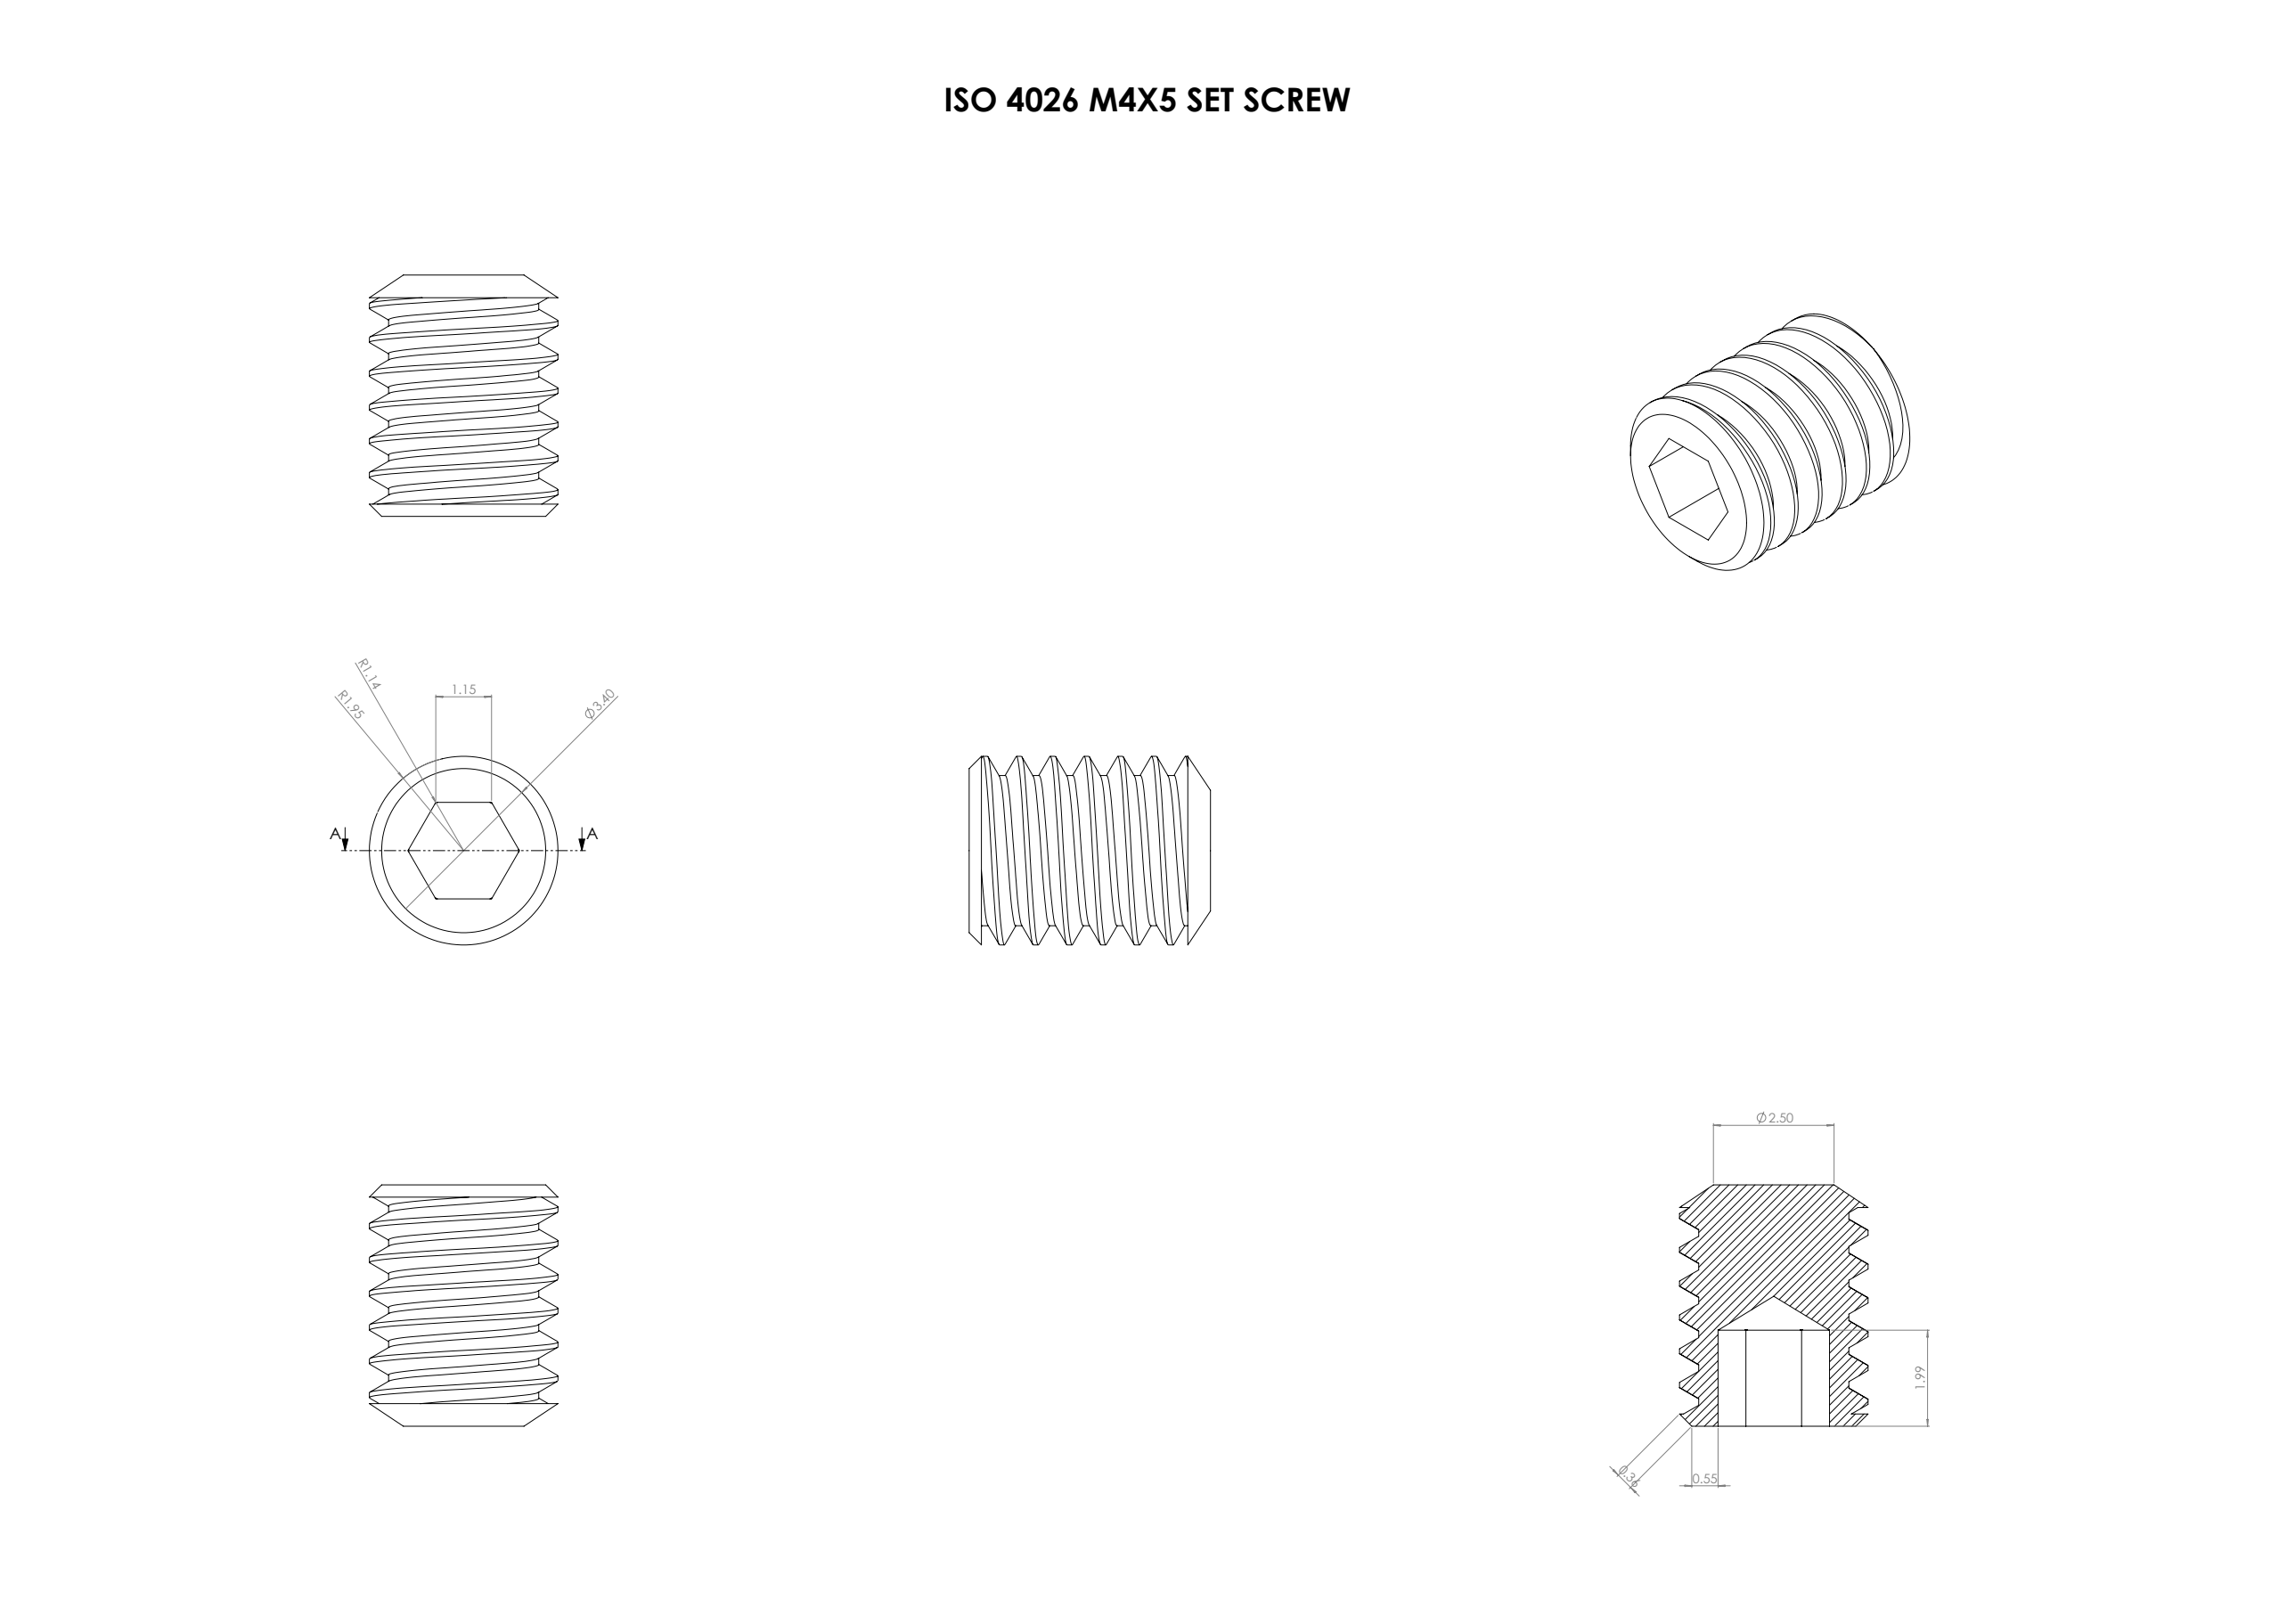
ISO-10303-21;
HEADER;
/* Generated by software containing ST-Developer
 * from STEP Tools, Inc. (www.steptools.com) 
 */

FILE_DESCRIPTION(
/* description */ (''),
/* implementation_level */ '2;1');

FILE_NAME(
/* name */ 
'13_ISO_4026_M4x5_Set_Screw.step',
/* time_stamp */ '2026-10-20T10:06:23-07:00',
/* author */ (''),
/* organization */ (''),
/* preprocessor_version */ 'ST-DEVELOPER v20.2',
/* originating_system */ 'Autodesk Translation Framework v15.15.0.0',
/* authorisation */ '');

FILE_SCHEMA (('AUTOMOTIVE_DESIGN { 1 0 10303 214 3 1 1 }'));
ENDSEC;

DATA;
#10=MECHANICAL_DESIGN_GEOMETRIC_PRESENTATION_REPRESENTATION('',(#466),#38611);
#106=(
BOUNDED_CURVE()
B_SPLINE_CURVE(2,(#25662,#25663,#25664),.UNSPECIFIED.,.F.,.F.)
B_SPLINE_CURVE_WITH_KNOTS((3,3),(0.,0.00350597452849922),.UNSPECIFIED.)
CURVE()
GEOMETRIC_REPRESENTATION_ITEM()
RATIONAL_B_SPLINE_CURVE((1.,1.00010739978215,1.))
REPRESENTATION_ITEM('')
);
#107=(
BOUNDED_CURVE()
B_SPLINE_CURVE(2,(#25666,#25667,#25668),.UNSPECIFIED.,.F.,.F.)
B_SPLINE_CURVE_WITH_KNOTS((3,3),(0.,0.00350597452849927),.UNSPECIFIED.)
CURVE()
GEOMETRIC_REPRESENTATION_ITEM()
RATIONAL_B_SPLINE_CURVE((1.,1.00010739978482,1.))
REPRESENTATION_ITEM('')
);
#108=(
BOUNDED_CURVE()
B_SPLINE_CURVE(2,(#25671,#25672,#25673),.UNSPECIFIED.,.F.,.F.)
B_SPLINE_CURVE_WITH_KNOTS((3,3),(0.,0.0035059745284993),.UNSPECIFIED.)
CURVE()
GEOMETRIC_REPRESENTATION_ITEM()
RATIONAL_B_SPLINE_CURVE((1.,1.00010739978303,1.))
REPRESENTATION_ITEM('')
);
#109=(
BOUNDED_CURVE()
B_SPLINE_CURVE(2,(#25675,#25676,#25677),.UNSPECIFIED.,.F.,.F.)
B_SPLINE_CURVE_WITH_KNOTS((3,3),(0.,0.00350597452849931),.UNSPECIFIED.)
CURVE()
GEOMETRIC_REPRESENTATION_ITEM()
RATIONAL_B_SPLINE_CURVE((1.,1.00010739978394,1.))
REPRESENTATION_ITEM('')
);
#110=(
BOUNDED_CURVE()
B_SPLINE_CURVE(2,(#25680,#25681,#25682),.UNSPECIFIED.,.F.,.F.)
B_SPLINE_CURVE_WITH_KNOTS((3,3),(0.,0.0035059745284993),.UNSPECIFIED.)
CURVE()
GEOMETRIC_REPRESENTATION_ITEM()
RATIONAL_B_SPLINE_CURVE((1.,1.00010739978631,1.))
REPRESENTATION_ITEM('')
);
#111=(
BOUNDED_CURVE()
B_SPLINE_CURVE(2,(#25684,#25685,#25686),.UNSPECIFIED.,.F.,.F.)
B_SPLINE_CURVE_WITH_KNOTS((3,3),(0.,0.00350597452849929),.UNSPECIFIED.)
CURVE()
GEOMETRIC_REPRESENTATION_ITEM()
RATIONAL_B_SPLINE_CURVE((1.,1.00010739978645,1.))
REPRESENTATION_ITEM('')
);
#112=(
BOUNDED_CURVE()
B_SPLINE_CURVE(2,(#25689,#25690,#25691),.UNSPECIFIED.,.F.,.F.)
B_SPLINE_CURVE_WITH_KNOTS((3,3),(0.,0.0035059745284993),.UNSPECIFIED.)
CURVE()
GEOMETRIC_REPRESENTATION_ITEM()
RATIONAL_B_SPLINE_CURVE((1.,1.00010739979569,1.))
REPRESENTATION_ITEM('')
);
#113=(
BOUNDED_CURVE()
B_SPLINE_CURVE(2,(#25693,#25694,#25695),.UNSPECIFIED.,.F.,.F.)
B_SPLINE_CURVE_WITH_KNOTS((3,3),(0.,0.0035059745284993),.UNSPECIFIED.)
CURVE()
GEOMETRIC_REPRESENTATION_ITEM()
RATIONAL_B_SPLINE_CURVE((1.,1.00010739979698,1.))
REPRESENTATION_ITEM('')
);
#114=(
BOUNDED_CURVE()
B_SPLINE_CURVE(2,(#25698,#25699,#25700),.UNSPECIFIED.,.F.,.F.)
B_SPLINE_CURVE_WITH_KNOTS((3,3),(0.,0.00350597452849928),.UNSPECIFIED.)
CURVE()
GEOMETRIC_REPRESENTATION_ITEM()
RATIONAL_B_SPLINE_CURVE((1.,1.00010739978256,1.))
REPRESENTATION_ITEM('')
);
#115=(
BOUNDED_CURVE()
B_SPLINE_CURVE(2,(#25702,#25703,#25704),.UNSPECIFIED.,.F.,.F.)
B_SPLINE_CURVE_WITH_KNOTS((3,3),(0.,0.00350597452849928),.UNSPECIFIED.)
CURVE()
GEOMETRIC_REPRESENTATION_ITEM()
RATIONAL_B_SPLINE_CURVE((1.,1.00010739978752,1.))
REPRESENTATION_ITEM('')
);
#116=(
BOUNDED_CURVE()
B_SPLINE_CURVE(2,(#25707,#25708,#25709),.UNSPECIFIED.,.F.,.F.)
B_SPLINE_CURVE_WITH_KNOTS((3,3),(0.,0.0035059745284993),.UNSPECIFIED.)
CURVE()
GEOMETRIC_REPRESENTATION_ITEM()
RATIONAL_B_SPLINE_CURVE((1.,1.0001073997843,1.))
REPRESENTATION_ITEM('')
);
#117=(
BOUNDED_CURVE()
B_SPLINE_CURVE(2,(#25711,#25712,#25713),.UNSPECIFIED.,.F.,.F.)
B_SPLINE_CURVE_WITH_KNOTS((3,3),(0.,0.00350597452849929),.UNSPECIFIED.)
CURVE()
GEOMETRIC_REPRESENTATION_ITEM()
RATIONAL_B_SPLINE_CURVE((1.,1.00010739978875,1.))
REPRESENTATION_ITEM('')
);
#438=SHAPE_REPRESENTATION_RELATIONSHIP('SRR','None',#38674,#452);
#452=ADVANCED_BREP_SHAPE_REPRESENTATION('',(#480),#38603);
#466=STYLED_ITEM('',(#38885),#480);
#480=MANIFOLD_SOLID_BREP('Set screw',#16240);
#497=B_SPLINE_SURFACE_WITH_KNOTS('',3,3,((#25107,#25108,#25109,#25110,#25111,
#25112,#25113,#25114,#25115,#25116,#25117,#25118,#25119,#25120,#25121,#25122,
#25123,#25124,#25125,#25126,#25127,#25128,#25129,#25130,#25131,#25132,#25133,
#25134,#25135,#25136,#25137,#25138,#25139,#25140,#25141,#25142,#25143,#25144,
#25145,#25146,#25147,#25148,#25149,#25150),(#25151,#25152,#25153,#25154,
#25155,#25156,#25157,#25158,#25159,#25160,#25161,#25162,#25163,#25164,#25165,
#25166,#25167,#25168,#25169,#25170,#25171,#25172,#25173,#25174,#25175,#25176,
#25177,#25178,#25179,#25180,#25181,#25182,#25183,#25184,#25185,#25186,#25187,
#25188,#25189,#25190,#25191,#25192,#25193,#25194),(#25195,#25196,#25197,
#25198,#25199,#25200,#25201,#25202,#25203,#25204,#25205,#25206,#25207,#25208,
#25209,#25210,#25211,#25212,#25213,#25214,#25215,#25216,#25217,#25218,#25219,
#25220,#25221,#25222,#25223,#25224,#25225,#25226,#25227,#25228,#25229,#25230,
#25231,#25232,#25233,#25234,#25235,#25236,#25237,#25238),(#25239,#25240,
#25241,#25242,#25243,#25244,#25245,#25246,#25247,#25248,#25249,#25250,#25251,
#25252,#25253,#25254,#25255,#25256,#25257,#25258,#25259,#25260,#25261,#25262,
#25263,#25264,#25265,#25266,#25267,#25268,#25269,#25270,#25271,#25272,#25273,
#25274,#25275,#25276,#25277,#25278,#25279,#25280,#25281,#25282)),
 .UNSPECIFIED.,.F.,.F.,.F.,(4,4),(4,1,1,1,1,1,1,1,1,1,1,1,1,1,1,1,1,1,1,
1,1,1,1,1,1,1,1,1,1,1,1,1,1,1,1,1,1,1,1,1,1,4),(0.,0.0460148164544132),
(8.31058692273977,9.29723107803592,10.2838752333321,11.2705193886282,12.2571635439244,
13.2438076992205,14.2304518545166,15.2170960098128,16.2037401651089,17.1903843204051,
18.1770284757012,19.1636726309974,20.1503167862935,21.1369609415897,22.1236050968858,
23.110249252182,24.0968934074781,25.0835375627742,26.0701817180704,27.0568258733665,
28.0434700286627,29.0301141839588,30.016758339255,31.0034024945511,31.9900466498473,
32.9766908051434,33.9633349604396,34.9499791157357,35.9366232710318,36.923267426328,
37.9099115816241,38.8965557369203,39.8831998922164,40.8698440475126,41.8564882028087,
42.8431323581049,43.829776513401,44.8164206686971,45.8030648239933,46.7897089792894,
47.7763531345856,48.7629972898817),.UNSPECIFIED.);
#498=B_SPLINE_SURFACE_WITH_KNOTS('',3,3,((#25437,#25438,#25439,#25440,#25441,
#25442,#25443,#25444,#25445,#25446,#25447,#25448,#25449,#25450,#25451,#25452,
#25453,#25454,#25455,#25456,#25457,#25458,#25459,#25460,#25461,#25462,#25463,
#25464,#25465,#25466,#25467,#25468,#25469,#25470,#25471,#25472,#25473,#25474,
#25475,#25476,#25477,#25478,#25479,#25480),(#25481,#25482,#25483,#25484,
#25485,#25486,#25487,#25488,#25489,#25490,#25491,#25492,#25493,#25494,#25495,
#25496,#25497,#25498,#25499,#25500,#25501,#25502,#25503,#25504,#25505,#25506,
#25507,#25508,#25509,#25510,#25511,#25512,#25513,#25514,#25515,#25516,#25517,
#25518,#25519,#25520,#25521,#25522,#25523,#25524),(#25525,#25526,#25527,
#25528,#25529,#25530,#25531,#25532,#25533,#25534,#25535,#25536,#25537,#25538,
#25539,#25540,#25541,#25542,#25543,#25544,#25545,#25546,#25547,#25548,#25549,
#25550,#25551,#25552,#25553,#25554,#25555,#25556,#25557,#25558,#25559,#25560,
#25561,#25562,#25563,#25564,#25565,#25566,#25567,#25568),(#25569,#25570,
#25571,#25572,#25573,#25574,#25575,#25576,#25577,#25578,#25579,#25580,#25581,
#25582,#25583,#25584,#25585,#25586,#25587,#25588,#25589,#25590,#25591,#25592,
#25593,#25594,#25595,#25596,#25597,#25598,#25599,#25600,#25601,#25602,#25603,
#25604,#25605,#25606,#25607,#25608,#25609,#25610,#25611,#25612)),
 .UNSPECIFIED.,.F.,.F.,.F.,(4,4),(4,1,1,1,1,1,1,1,1,1,1,1,1,1,1,1,1,1,1,
1,1,1,1,1,1,1,1,1,1,1,1,1,1,1,1,1,1,1,1,1,1,4),(0.,0.0460148164544132),
(11.6154215191106,12.6020656744068,13.5887098297029,14.5753539849991,15.5619981402952,
16.5486422955914,17.5352864508875,18.5219306061837,19.5085747614798,20.4952189167759,
21.4818630720721,22.4685072273682,23.4551513826644,24.4417955379605,25.4284396932567,
26.4150838485528,27.401728003849,28.3883721591451,29.3750163144413,30.3616604697374,
31.3483046250335,32.3349487803297,33.3215929356258,34.308237090922,35.2948812462181,
36.2815254015143,37.2681695568104,38.2548137121066,39.2414578674027,40.2281020226988,
41.214746177995,42.2013903332911,43.1880344885873,44.1746786438834,45.1613227991796,
46.1479669544757,47.1346111097719,48.121255265068,49.1078994203642,50.0945435756603,
51.0811877309565,52.0678318862526),.UNSPECIFIED.);
#560=B_SPLINE_CURVE_WITH_KNOTS('',3,(#24587,#24588,#24589,#24590,#24591,
#24592,#24593,#24594,#24595,#24596),.UNSPECIFIED.,.F.,.F.,(4,3,3,4),(-4.09254174883832,
-3.94657662118458,-2.95993246588844,-2.06514013327811),.UNSPECIFIED.);
#561=B_SPLINE_CURVE_WITH_KNOTS('',3,(#24599,#24600,#24601,#24602,#24603,
#24604,#24605),.UNSPECIFIED.,.F.,.F.,(4,3,4),(0.,0.986644155296146,1.11419103802958),
 .UNSPECIFIED.);
#562=B_SPLINE_CURVE_WITH_KNOTS('',3,(#24610,#24611,#24612,#24613,#24614,
#24615,#24616,#24617,#24618,#24619,#24620,#24621,#24622,#24623,#24624,#24625,
#24626,#24627,#24628,#24629,#24630,#24631),.UNSPECIFIED.,.F.,.F.,(4,3,3,
3,3,3,3,4),(-10.3757270560179,-9.86644155296145,-8.87979739766531,-7.89315324236916,
-6.90650908707302,-5.91986493177687,-4.93322077648073,-4.09254174883832),
 .UNSPECIFIED.);
#563=B_SPLINE_CURVE_WITH_KNOTS('',3,(#24632,#24633,#24634,#24635,#24636,
#24637,#24638,#24639,#24640,#24641,#24642,#24643,#24644,#24645,#24646,#24647,
#24648,#24649,#24650,#24651,#24652,#24653),.UNSPECIFIED.,.F.,.F.,(4,3,3,
3,3,3,3,4),(1.11419103802958,1.97328831059229,2.95993246588844,3.94657662118458,
4.93322077648073,5.91986493177687,6.90650908707302,7.39737634520917),
 .UNSPECIFIED.);
#564=B_SPLINE_CURVE_WITH_KNOTS('',3,(#24658,#24659,#24660,#24661,#24662,
#24663,#24664,#24665,#24666,#24667,#24668,#24669,#24670,#24671,#24672,#24673,
#24674,#24675,#24676,#24677,#24678,#24679),.UNSPECIFIED.,.F.,.F.,(4,3,3,
3,3,3,3,4),(-16.6589123631975,-15.7863064847383,-14.7996623294422,-13.813018174146,
-12.8263740188499,-11.8397298635537,-10.8530857082576,-10.3757270560179),
 .UNSPECIFIED.);
#565=B_SPLINE_CURVE_WITH_KNOTS('',3,(#24680,#24681,#24682,#24683,#24684,
#24685,#24686,#24687,#24688,#24689,#24690,#24691,#24692,#24693,#24694,#24695,
#24696,#24697,#24698,#24699,#24700,#24701),.UNSPECIFIED.,.F.,.F.,(4,3,3,
3,3,3,3,4),(7.39737634520917,7.89315324236916,8.87979739766531,9.86644155296146,
10.8530857082576,11.8397298635537,12.8263740188499,13.6805616523888),
 .UNSPECIFIED.);
#566=B_SPLINE_CURVE_WITH_KNOTS('',3,(#24706,#24707,#24708,#24709,#24710,
#24711,#24712,#24713,#24714,#24715,#24716,#24717,#24718,#24719,#24720,#24721,
#24722,#24723,#24724,#24725,#24726,#24727,#24728,#24729,#24730),
 .UNSPECIFIED.,.F.,.F.,(4,3,3,3,3,3,3,3,4),(-22.9420976703771,-22.6928155718113,
-21.7061714165152,-20.719527261219,-19.7328831059229,-18.7462389506268,
-17.7595947953306,-16.7729506400345,-16.6589123631975),.UNSPECIFIED.);
#567=B_SPLINE_CURVE_WITH_KNOTS('',3,(#24731,#24732,#24733,#24734,#24735,
#24736,#24737,#24738,#24739,#24740,#24741,#24742,#24743,#24744,#24745,#24746,
#24747,#24748,#24749,#24750,#24751,#24752,#24753,#24754,#24755),
 .UNSPECIFIED.,.F.,.F.,(4,3,3,3,3,3,3,3,4),(13.6805616523888,13.813018174146,
14.7996623294422,15.7863064847383,16.7729506400345,17.7595947953306,18.7462389506268,
19.7328831059229,19.9637469595683),.UNSPECIFIED.);
#568=B_SPLINE_CURVE_WITH_KNOTS('',3,(#24760,#24761,#24762,#24763,#24764,
#24765,#24766,#24767,#24768,#24769,#24770,#24771,#24772,#24773,#24774,#24775,
#24776,#24777,#24778,#24779,#24780,#24781),.UNSPECIFIED.,.F.,.F.,(4,3,3,
3,3,3,3,4),(-29.2252829775567,-28.6126805035882,-27.6260363482921,-26.6393921929959,
-25.6527480376998,-24.6661038824036,-23.6794597271075,-22.9420976703771),
 .UNSPECIFIED.);
#569=B_SPLINE_CURVE_WITH_KNOTS('',3,(#24782,#24783,#24784,#24785,#24786,
#24787,#24788,#24789,#24790,#24791,#24792,#24793,#24794,#24795,#24796,#24797,
#24798,#24799,#24800,#24801,#24802,#24803),.UNSPECIFIED.,.F.,.F.,(4,3,3,
3,3,3,3,4),(19.9637469595683,20.719527261219,21.7061714165152,22.6928155718113,
23.6794597271075,24.6661038824036,25.6527480376998,26.2469322667479),
 .UNSPECIFIED.);
#570=B_SPLINE_CURVE_WITH_KNOTS('',3,(#24808,#24809,#24810,#24811,#24812,
#24813,#24814,#24815,#24816,#24817,#24818,#24819,#24820,#24821,#24822,#24823,
#24824,#24825,#24826,#24827,#24828,#24829),.UNSPECIFIED.,.F.,.F.,(4,3,3,
3,3,3,3,4),(-35.5084682847363,-34.5325454353651,-33.5459012800689,-32.5592571247728,
-31.5726129694767,-30.5859688141805,-29.5993246588844,-29.2252829775567),
 .UNSPECIFIED.);
#571=B_SPLINE_CURVE_WITH_KNOTS('',3,(#24830,#24831,#24832,#24833,#24834,
#24835,#24836,#24837,#24838,#24839,#24840,#24841,#24842,#24843,#24844,#24845,
#24846,#24847,#24848,#24849,#24850,#24851),.UNSPECIFIED.,.F.,.F.,(4,3,3,
3,3,3,3,4),(26.2469322667479,26.6393921929959,27.6260363482921,28.6126805035882,
29.5993246588844,30.5859688141805,31.5726129694767,32.5301175739275),
 .UNSPECIFIED.);
#572=B_SPLINE_CURVE_WITH_KNOTS('',3,(#24857,#24858,#24859,#24860,#24861,
#24862,#24863),.UNSPECIFIED.,.F.,.F.,(4,1,1,1,4),(47.1238898038469,47.1346111097719,
48.121255265068,49.1078994203642,50.0026917529745),.UNSPECIFIED.);
#573=B_SPLINE_CURVE_WITH_KNOTS('',3,(#24866,#24867,#24868,#24869,#24870),
 .UNSPECIFIED.,.F.,.F.,(4,1,4),(47.1238898038469,47.7763531345856,48.7629972898817),
 .UNSPECIFIED.);
#574=B_SPLINE_CURVE_WITH_KNOTS('',3,(#24875,#24876,#24877,#24878,#24879,
#24880,#24881,#24882,#24883,#24884),.UNSPECIFIED.,.F.,.F.,(4,1,1,1,1,1,
1,4),(40.8407044966673,41.214746177995,42.2013903332911,43.1880344885873,
44.1746786438834,45.1613227991796,46.1479669544757,47.1238898038469),
 .UNSPECIFIED.);
#575=B_SPLINE_CURVE_WITH_KNOTS('',3,(#24885,#24886,#24887,#24888,#24889,
#24890,#24891,#24892,#24893,#24894,#24895),.UNSPECIFIED.,.F.,.F.,(4,1,1,
1,1,1,1,1,4),(40.8407044966673,40.8698440475126,41.8564882028087,42.8431323581049,
43.829776513401,44.8164206686971,45.8030648239933,46.7897089792894,47.1238898038469),
 .UNSPECIFIED.);
#576=B_SPLINE_CURVE_WITH_KNOTS('',3,(#24900,#24901,#24902,#24903,#24904,
#24905,#24906,#24907,#24908,#24909),.UNSPECIFIED.,.F.,.F.,(4,1,1,1,1,1,
1,4),(34.5575191894877,35.2948812462181,36.2815254015143,37.2681695568104,
38.2548137121066,39.2414578674027,40.2281020226988,40.8407044966673),
 .UNSPECIFIED.);
#577=B_SPLINE_CURVE_WITH_KNOTS('',3,(#24910,#24911,#24912,#24913,#24914,
#24915,#24916,#24917,#24918,#24919),.UNSPECIFIED.,.F.,.F.,(4,1,1,1,1,1,
1,4),(34.5575191894877,34.9499791157357,35.9366232710318,36.923267426328,
37.9099115816241,38.8965557369203,39.8831998922164,40.8407044966673),
 .UNSPECIFIED.);
#578=B_SPLINE_CURVE_WITH_KNOTS('',3,(#24924,#24925,#24926,#24927,#24928,
#24929,#24930,#24931,#24932,#24933,#24934),.UNSPECIFIED.,.F.,.F.,(4,1,1,
1,1,1,1,1,4),(28.2743338823081,28.3883721591451,29.3750163144413,30.3616604697374,
31.3483046250335,32.3349487803297,33.3215929356258,34.308237090922,34.5575191894877),
 .UNSPECIFIED.);
#579=B_SPLINE_CURVE_WITH_KNOTS('',3,(#24935,#24936,#24937,#24938,#24939,
#24940,#24941,#24942,#24943,#24944),.UNSPECIFIED.,.F.,.F.,(4,1,1,1,1,1,
1,4),(28.2743338823081,29.0301141839588,30.016758339255,31.0034024945511,
31.9900466498473,32.9766908051434,33.9633349604396,34.5575191894877),
 .UNSPECIFIED.);
#580=B_SPLINE_CURVE_WITH_KNOTS('',3,(#24949,#24950,#24951,#24952,#24953,
#24954,#24955,#24956,#24957,#24958),.UNSPECIFIED.,.F.,.F.,(4,1,1,1,1,1,
1,4),(21.9911485751285,22.4685072273682,23.4551513826644,24.4417955379605,
25.4284396932567,26.4150838485528,27.401728003849,28.2743338823081),
 .UNSPECIFIED.);
#581=B_SPLINE_CURVE_WITH_KNOTS('',3,(#24959,#24960,#24961,#24962,#24963,
#24964,#24965,#24966,#24967,#24968,#24969),.UNSPECIFIED.,.F.,.F.,(4,1,1,
1,1,1,1,1,4),(21.9911485751285,22.1236050968858,23.110249252182,24.0968934074781,
25.0835375627742,26.0701817180704,27.0568258733665,28.0434700286627,28.2743338823081),
 .UNSPECIFIED.);
#582=B_SPLINE_CURVE_WITH_KNOTS('',3,(#24974,#24975,#24976,#24977,#24978,
#24979,#24980,#24981,#24982,#24983),.UNSPECIFIED.,.F.,.F.,(4,1,1,1,1,1,
1,4),(15.707963267949,16.5486422955914,17.5352864508875,18.5219306061837,
19.5085747614798,20.4952189167759,21.4818630720721,21.9911485751285),
 .UNSPECIFIED.);
#583=B_SPLINE_CURVE_WITH_KNOTS('',3,(#24984,#24985,#24986,#24987,#24988,
#24989,#24990,#24991,#24992,#24993),.UNSPECIFIED.,.F.,.F.,(4,1,1,1,1,1,
1,4),(15.7079632679489,16.2037401651089,17.1903843204051,18.1770284757012,
19.1636726309974,20.1503167862935,21.1369609415897,21.9911485751285),
 .UNSPECIFIED.);
#584=B_SPLINE_CURVE_WITH_KNOTS('',3,(#24996,#24997,#24998,#24999,#25000,
#25001,#25002,#25003,#25004,#25005,#25006,#25007,#25008,#25009,#25010,#25011,
#25012,#25013,#25014,#25015,#25016,#25017,#25018,#25019,#25020,#25021,#25022,
#25023,#25024,#25025,#25026,#25027,#25028,#25029,#25030,#25031,#25032,#25033,
#25034,#25035,#25036,#25037,#25038,#25039,#25040,#25041,#25042,#25043,#25044,
#25045,#25046,#25047),.UNSPECIFIED.,.F.,.F.,(4,3,3,3,3,3,3,3,3,3,3,3,3,
3,3,3,3,4),(-0.366397579005847,-0.351842688178875,-0.332838158855069,-0.315678481693382,
-0.289420321645097,-0.273011785342624,-0.237897749313856,-0.221715923866805,
-0.207723971026893,-0.185180840167277,-0.161636550067305,-0.147128811889025,
-0.135731814711402,-0.101798861033552,-0.076880688176872,-0.0670092782892109,
-0.0285139790106868,0.),.UNSPECIFIED.);
#585=B_SPLINE_CURVE_WITH_KNOTS('',3,(#25052,#25053,#25054,#25055,#25056,
#25057,#25058,#25059,#25060,#25061,#25062,#25063,#25064,#25065,#25066,#25067,
#25068,#25069,#25070,#25071,#25072,#25073,#25074,#25075,#25076,#25077,#25078,
#25079,#25080,#25081,#25082,#25083,#25084,#25085,#25086,#25087,#25088,#25089,
#25090,#25091,#25092,#25093,#25094,#25095,#25096,#25097,#25098,#25099,#25100,
#25101,#25102,#25103,#25104,#25105,#25106),.UNSPECIFIED.,.F.,.F.,(4,3,3,
3,3,3,3,3,3,3,3,3,3,3,3,3,3,3,4),(-0.364629307890685,-0.346730130939237,
-0.318258076668756,-0.304671300367645,-0.283283926727407,-0.268750032662776,
-0.256211185988777,-0.219678588916904,-0.20148985221534,-0.1862389075973,
-0.164290383513372,-0.139072476943319,-0.127435374126706,-0.116240718055298,
-0.0871805385414733,-0.0683502117761216,-0.0546744719449251,-0.022336513706662,
0.),.UNSPECIFIED.);
#586=B_SPLINE_CURVE_WITH_KNOTS('',3,(#25283,#25284,#25285,#25286,#25287,
#25288,#25289,#25290,#25291,#25292,#25293,#25294,#25295,#25296,#25297,#25298,
#25299,#25300,#25301,#25302,#25303,#25304),.UNSPECIFIED.,.F.,.F.,(4,3,3,
3,3,3,3,4),(32.5301175739275,32.5592571247728,33.5459012800689,34.5325454353651,
35.5191895906612,36.5058337459574,37.4924779012535,38.3872702338639),
 .UNSPECIFIED.);
#587=B_SPLINE_CURVE_WITH_KNOTS('',3,(#25306,#25307,#25308,#25309,#25310,
#25311,#25312,#25313,#25314,#25315,#25316,#25317,#25318,#25319,#25320,#25321,
#25322,#25323,#25324,#25325,#25326,#25327,#25328,#25329,#25330,#25331,#25332,
#25333,#25334,#25335,#25336,#25337,#25338,#25339,#25340,#25341,#25342,#25343,
#25344,#25345,#25346,#25347,#25348,#25349,#25350,#25351,#25352,#25353,#25354,
#25355,#25356,#25357),.UNSPECIFIED.,.F.,.F.,(4,3,3,3,3,3,3,3,3,3,3,3,3,
3,3,3,3,4),(-0.36639757900584,-0.351842688178868,-0.332838163030847,-0.315678486081905,
-0.289414746484995,-0.273012692426124,-0.237898677161377,-0.221717024761523,
-0.207724021339265,-0.18518084016727,-0.161636547239729,-0.147128781690345,
-0.135731805846515,-0.101798854384886,-0.0768806612204703,-0.0670092358876265,
-0.0285139219945927,0.),.UNSPECIFIED.);
#588=B_SPLINE_CURVE_WITH_KNOTS('',3,(#25358,#25359,#25360,#25361,#25362,
#25363,#25364,#25365,#25366),.UNSPECIFIED.,.F.,.F.,(4,1,1,1,1,1,4),(10.3757270560179,
11.2705193886282,12.2571635439244,13.2438076992205,14.2304518545166,15.2170960098128,
15.7079632679489),.UNSPECIFIED.);
#589=B_SPLINE_CURVE_WITH_KNOTS('',3,(#25372,#25373,#25374,#25375,#25376,
#25377,#25378,#25379,#25380,#25381,#25382,#25383,#25384,#25385,#25386,#25387,
#25388,#25389,#25390,#25391,#25392,#25393,#25394,#25395,#25396,#25397,#25398,
#25399,#25400,#25401,#25402,#25403,#25404,#25405,#25406,#25407,#25408,#25409,
#25410,#25411,#25412,#25413,#25414,#25415,#25416,#25417,#25418,#25419,#25420,
#25421,#25422,#25423,#25424,#25425,#25426),.UNSPECIFIED.,.F.,.F.,(4,3,3,
3,3,3,3,3,3,3,3,3,3,3,3,3,3,3,4),(-0.36462930789067,-0.346730130939223,
-0.318258061840929,-0.304671288555113,-0.283283871503023,-0.268749409502959,
-0.256211230718671,-0.219678613621225,-0.201489854814136,-0.186238903270344,
-0.164290383513369,-0.139072549937506,-0.127435742460392,-0.116240765389693,
-0.0871805740422699,-0.0683502946375612,-0.0546744738896406,-0.0223365680991636,
0.),.UNSPECIFIED.);
#590=B_SPLINE_CURVE_WITH_KNOTS('',3,(#25429,#25430,#25431,#25432,#25433,
#25434,#25435,#25436),.UNSPECIFIED.,.F.,.F.,(4,1,1,1,1,4),(11.6154215191106,
12.6020656744068,13.5887098297029,14.5753539849991,15.5619981402952,15.707963267949),
 .UNSPECIFIED.);
#591=B_SPLINE_CURVE_WITH_KNOTS('',3,(#25613,#25614,#25615,#25616,#25617,
#25618,#25619,#25620,#25621,#25622,#25623,#25624,#25625,#25626,#25627,#25628,
#25629,#25630,#25631),.UNSPECIFIED.,.F.,.F.,(4,3,3,3,3,3,4),(-40.452410367142,
-39.4657662118458,-38.4791220565497,-37.4924779012535,-36.5058337459574,
-35.5191895906612,-35.5084682847363),.UNSPECIFIED.);
#916=CYLINDRICAL_SURFACE('',#16835,0.1954);
#917=CYLINDRICAL_SURFACE('',#16837,0.1954);
#918=CYLINDRICAL_SURFACE('',#16838,0.1954);
#919=CYLINDRICAL_SURFACE('',#16839,0.1954);
#920=CYLINDRICAL_SURFACE('',#16840,0.1954);
#921=CYLINDRICAL_SURFACE('',#16841,0.1954);
#922=CYLINDRICAL_SURFACE('',#16842,0.15555);
#923=CYLINDRICAL_SURFACE('',#16844,0.15555);
#924=CYLINDRICAL_SURFACE('',#16845,0.15555);
#925=CYLINDRICAL_SURFACE('',#16846,0.15555);
#926=CYLINDRICAL_SURFACE('',#16847,0.15555);
#927=CYLINDRICAL_SURFACE('',#16848,0.15555);
#928=CYLINDRICAL_SURFACE('',#16856,0.15555);
#929=CYLINDRICAL_SURFACE('',#16904,0.1954);
#1186=FACE_BOUND('',#3044,.T.);
#1363=CIRCLE('',#16836,0.1954);
#1364=CIRCLE('',#16843,0.15555);
#1365=CIRCLE('',#16850,0.1954);
#1366=CIRCLE('',#16851,0.1954);
#1367=CIRCLE('',#16853,0.1954);
#1368=CIRCLE('',#16854,0.1954);
#1369=CIRCLE('',#16855,0.15555);
#1370=CIRCLE('',#16858,0.115470053837925);
#1371=CIRCLE('',#16860,0.115470053837925);
#1372=CIRCLE('',#16862,0.115470053837925);
#1373=CIRCLE('',#16864,0.115470053837925);
#1374=CIRCLE('',#16866,0.115470053837925);
#1375=CIRCLE('',#16868,0.115470053837925);
#1376=CIRCLE('',#16870,0.113827101150665);
#1377=CIRCLE('',#16871,0.113827101150665);
#1378=CIRCLE('',#16872,0.113827101150665);
#1379=CIRCLE('',#16873,0.113827101150665);
#1380=CIRCLE('',#16874,0.113827101150665);
#1381=CIRCLE('',#16875,0.113827101150665);
#1382=CIRCLE('',#16876,0.113827101150665);
#1383=CIRCLE('',#16902,0.125);
#1384=CIRCLE('',#16905,0.1954);
#1385=CIRCLE('',#16907,0.17);
#1740=CONICAL_SURFACE('',#16869,0.0577350269189626,1.02403331474479);
#1741=CONICAL_SURFACE('',#16903,0.1625,0.982793723247329);
#1742=CONICAL_SURFACE('',#16906,0.185,0.785398163397449);
#2047=FACE_OUTER_BOUND('',#2991,.T.);
#2048=FACE_OUTER_BOUND('',#2992,.T.);
#2049=FACE_OUTER_BOUND('',#2993,.T.);
#2050=FACE_OUTER_BOUND('',#2994,.T.);
#2051=FACE_OUTER_BOUND('',#2995,.T.);
#2052=FACE_OUTER_BOUND('',#2996,.T.);
#2053=FACE_OUTER_BOUND('',#2997,.T.);
#2054=FACE_OUTER_BOUND('',#2998,.T.);
#2055=FACE_OUTER_BOUND('',#2999,.T.);
#2056=FACE_OUTER_BOUND('',#3000,.T.);
#2057=FACE_OUTER_BOUND('',#3001,.T.);
#2058=FACE_OUTER_BOUND('',#3002,.T.);
#2059=FACE_OUTER_BOUND('',#3003,.T.);
#2060=FACE_OUTER_BOUND('',#3004,.T.);
#2061=FACE_OUTER_BOUND('',#3005,.T.);
#2062=FACE_OUTER_BOUND('',#3006,.T.);
#2063=FACE_OUTER_BOUND('',#3007,.T.);
#2064=FACE_OUTER_BOUND('',#3008,.T.);
#2065=FACE_OUTER_BOUND('',#3009,.T.);
#2066=FACE_OUTER_BOUND('',#3010,.T.);
#2067=FACE_OUTER_BOUND('',#3011,.T.);
#2068=FACE_OUTER_BOUND('',#3012,.T.);
#2069=FACE_OUTER_BOUND('',#3013,.T.);
#2070=FACE_OUTER_BOUND('',#3014,.T.);
#2071=FACE_OUTER_BOUND('',#3015,.T.);
#2072=FACE_OUTER_BOUND('',#3016,.T.);
#2073=FACE_OUTER_BOUND('',#3017,.T.);
#2074=FACE_OUTER_BOUND('',#3018,.T.);
#2075=FACE_OUTER_BOUND('',#3019,.T.);
#2076=FACE_OUTER_BOUND('',#3020,.T.);
#2077=FACE_OUTER_BOUND('',#3021,.T.);
#2078=FACE_OUTER_BOUND('',#3022,.T.);
#2079=FACE_OUTER_BOUND('',#3023,.T.);
#2080=FACE_OUTER_BOUND('',#3024,.T.);
#2081=FACE_OUTER_BOUND('',#3025,.T.);
#2082=FACE_OUTER_BOUND('',#3026,.T.);
#2083=FACE_OUTER_BOUND('',#3027,.T.);
#2084=FACE_OUTER_BOUND('',#3028,.T.);
#2085=FACE_OUTER_BOUND('',#3029,.T.);
#2086=FACE_OUTER_BOUND('',#3030,.T.);
#2087=FACE_OUTER_BOUND('',#3031,.T.);
#2088=FACE_OUTER_BOUND('',#3032,.T.);
#2089=FACE_OUTER_BOUND('',#3033,.T.);
#2090=FACE_OUTER_BOUND('',#3034,.T.);
#2091=FACE_OUTER_BOUND('',#3035,.T.);
#2092=FACE_OUTER_BOUND('',#3036,.T.);
#2093=FACE_OUTER_BOUND('',#3037,.T.);
#2094=FACE_OUTER_BOUND('',#3038,.T.);
#2095=FACE_OUTER_BOUND('',#3039,.T.);
#2096=FACE_OUTER_BOUND('',#3040,.T.);
#2097=FACE_OUTER_BOUND('',#3041,.T.);
#2098=FACE_OUTER_BOUND('',#3042,.T.);
#2099=FACE_OUTER_BOUND('',#3043,.T.);
#2991=EDGE_LOOP('',(#11365,#11366,#11367,#11368));
#2992=EDGE_LOOP('',(#11369,#11370,#11371,#11372));
#2993=EDGE_LOOP('',(#11373,#11374,#11375,#11376));
#2994=EDGE_LOOP('',(#11377,#11378,#11379,#11380));
#2995=EDGE_LOOP('',(#11381,#11382,#11383,#11384));
#2996=EDGE_LOOP('',(#11385,#11386,#11387,#11388));
#2997=EDGE_LOOP('',(#11389,#11390,#11391,#11392));
#2998=EDGE_LOOP('',(#11393,#11394,#11395,#11396));
#2999=EDGE_LOOP('',(#11397,#11398,#11399,#11400));
#3000=EDGE_LOOP('',(#11401,#11402,#11403,#11404));
#3001=EDGE_LOOP('',(#11405,#11406,#11407,#11408));
#3002=EDGE_LOOP('',(#11409,#11410,#11411,#11412));
#3003=EDGE_LOOP('',(#11413,#11414,#11415,#11416,#11417));
#3004=EDGE_LOOP('',(#11418,#11419,#11420,#11421,#11422,#11423,#11424,#11425,
#11426,#11427,#11428,#11429,#11430,#11431,#11432,#11433));
#3005=EDGE_LOOP('',(#11434,#11435,#11436,#11437,#11438));
#3006=EDGE_LOOP('',(#11439,#11440,#11441,#11442));
#3007=EDGE_LOOP('',(#11443,#11444,#11445,#11446,#11447,#11448,#11449,#11450,
#11451,#11452,#11453,#11454,#11455,#11456,#11457,#11458));
#3008=EDGE_LOOP('',(#11459,#11460));
#3009=EDGE_LOOP('',(#11461,#11462));
#3010=EDGE_LOOP('',(#11463,#11464));
#3011=EDGE_LOOP('',(#11465,#11466));
#3012=EDGE_LOOP('',(#11467,#11468));
#3013=EDGE_LOOP('',(#11469,#11470));
#3014=EDGE_LOOP('',(#11471,#11472,#11473,#11474,#11475,#11476,#11477,#11478,
#11479,#11480,#11481,#11482,#11483,#11484,#11485,#11486,#11487,#11488,#11489,
#11490,#11491,#11492,#11493,#11494,#11495,#11496,#11497));
#3015=EDGE_LOOP('',(#11498,#11499,#11500,#11501));
#3016=EDGE_LOOP('',(#11502,#11503,#11504));
#3017=EDGE_LOOP('',(#11505,#11506,#11507,#11508));
#3018=EDGE_LOOP('',(#11509,#11510,#11511));
#3019=EDGE_LOOP('',(#11512,#11513,#11514));
#3020=EDGE_LOOP('',(#11515,#11516,#11517,#11518));
#3021=EDGE_LOOP('',(#11519,#11520,#11521));
#3022=EDGE_LOOP('',(#11522,#11523,#11524,#11525));
#3023=EDGE_LOOP('',(#11526,#11527,#11528));
#3024=EDGE_LOOP('',(#11529,#11530,#11531));
#3025=EDGE_LOOP('',(#11532,#11533,#11534));
#3026=EDGE_LOOP('',(#11535,#11536,#11537));
#3027=EDGE_LOOP('',(#11538,#11539,#11540));
#3028=EDGE_LOOP('',(#11541,#11542,#11543));
#3029=EDGE_LOOP('',(#11544,#11545,#11546));
#3030=EDGE_LOOP('',(#11547,#11548,#11549,#11550));
#3031=EDGE_LOOP('',(#11551,#11552,#11553,#11554));
#3032=EDGE_LOOP('',(#11555,#11556,#11557));
#3033=EDGE_LOOP('',(#11558,#11559,#11560));
#3034=EDGE_LOOP('',(#11561,#11562,#11563));
#3035=EDGE_LOOP('',(#11564,#11565,#11566,#11567));
#3036=EDGE_LOOP('',(#11568,#11569,#11570));
#3037=EDGE_LOOP('',(#11571,#11572,#11573));
#3038=EDGE_LOOP('',(#11574,#11575,#11576));
#3039=EDGE_LOOP('',(#11577));
#3040=EDGE_LOOP('',(#11578,#11579,#11580,#11581,#11582,#11583));
#3041=EDGE_LOOP('',(#11584,#11585,#11586,#11587));
#3042=EDGE_LOOP('',(#11588,#11589,#11590,#11591,#11592,#11593));
#3043=EDGE_LOOP('',(#11594));
#3044=EDGE_LOOP('',(#11595,#11596,#11597,#11598,#11599,#11600));
#4111=LINE('',#24585,#5335);
#4112=LINE('',#24609,#5336);
#4113=LINE('',#24657,#5337);
#4114=LINE('',#24705,#5338);
#4115=LINE('',#24759,#5339);
#4116=LINE('',#24807,#5340);
#4117=LINE('',#24855,#5341);
#4118=LINE('',#24874,#5342);
#4119=LINE('',#24899,#5343);
#4120=LINE('',#24923,#5344);
#4121=LINE('',#24948,#5345);
#4122=LINE('',#24973,#5346);
#4123=LINE('',#25635,#5347);
#4124=LINE('',#25639,#5348);
#4125=LINE('',#25643,#5349);
#4126=LINE('',#25647,#5350);
#4127=LINE('',#25651,#5351);
#4128=LINE('',#25654,#5352);
#4129=LINE('',#25659,#5353);
#4130=LINE('',#25717,#5354);
#4131=LINE('',#25719,#5355);
#4132=LINE('',#25720,#5356);
#4133=LINE('',#25723,#5357);
#4134=LINE('',#25724,#5358);
#4135=LINE('',#25727,#5359);
#4136=LINE('',#25728,#5360);
#4137=LINE('',#25731,#5361);
#4138=LINE('',#25732,#5362);
#4139=LINE('',#25735,#5363);
#4140=LINE('',#25736,#5364);
#4141=LINE('',#25739,#5365);
#4142=LINE('',#25740,#5366);
#4143=LINE('',#25743,#5367);
#4144=LINE('',#25744,#5368);
#4145=LINE('',#25747,#5369);
#4146=LINE('',#25748,#5370);
#4147=LINE('',#25751,#5371);
#4148=LINE('',#25752,#5372);
#4149=LINE('',#25754,#5373);
#4150=LINE('',#25756,#5374);
#4151=LINE('',#25759,#5375);
#4152=LINE('',#25762,#5376);
#4153=LINE('',#25763,#5377);
#4154=LINE('',#25765,#5378);
#4155=LINE('',#25767,#5379);
#4156=LINE('',#25770,#5380);
#4157=LINE('',#25771,#5381);
#4158=LINE('',#25773,#5382);
#4159=LINE('',#25777,#5383);
#4160=LINE('',#25785,#5384);
#4161=LINE('',#25791,#5385);
#5335=VECTOR('',#19128,0.2);
#5336=VECTOR('',#19133,0.2);
#5337=VECTOR('',#19136,0.2);
#5338=VECTOR('',#19139,0.2);
#5339=VECTOR('',#19142,0.2);
#5340=VECTOR('',#19145,0.2);
#5341=VECTOR('',#19148,0.15555);
#5342=VECTOR('',#19153,0.15555);
#5343=VECTOR('',#19156,0.15555);
#5344=VECTOR('',#19159,0.15555);
#5345=VECTOR('',#19162,0.15555);
#5346=VECTOR('',#19165,0.15555);
#5347=VECTOR('',#19184,1.);
#5348=VECTOR('',#19189,1.);
#5349=VECTOR('',#19194,1.);
#5350=VECTOR('',#19199,1.);
#5351=VECTOR('',#19204,1.);
#5352=VECTOR('',#19209,1.);
#5353=VECTOR('',#19214,0.0577350269189626);
#5354=VECTOR('',#19231,1.);
#5355=VECTOR('',#19232,1.);
#5356=VECTOR('',#19233,1.);
#5357=VECTOR('',#19236,1.);
#5358=VECTOR('',#19237,1.);
#5359=VECTOR('',#19240,1.);
#5360=VECTOR('',#19241,1.);
#5361=VECTOR('',#19244,1.);
#5362=VECTOR('',#19245,1.);
#5363=VECTOR('',#19248,1.);
#5364=VECTOR('',#19249,1.);
#5365=VECTOR('',#19252,1.);
#5366=VECTOR('',#19253,1.);
#5367=VECTOR('',#19256,1.);
#5368=VECTOR('',#19257,1.);
#5369=VECTOR('',#19260,1.);
#5370=VECTOR('',#19261,1.);
#5371=VECTOR('',#19264,1.);
#5372=VECTOR('',#19265,1.);
#5373=VECTOR('',#19268,1.);
#5374=VECTOR('',#19271,1.);
#5375=VECTOR('',#19276,1.);
#5376=VECTOR('',#19279,1.);
#5377=VECTOR('',#19280,1.);
#5378=VECTOR('',#19283,1.);
#5379=VECTOR('',#19286,1.);
#5380=VECTOR('',#19289,1.);
#5381=VECTOR('',#19290,1.);
#5382=VECTOR('',#19293,1.);
#5383=VECTOR('',#19300,1.);
#5384=VECTOR('',#19313,0.1625);
#5385=VECTOR('',#19322,0.185);
#6521=VERTEX_POINT('',#24583);
#6522=VERTEX_POINT('',#24584);
#6523=VERTEX_POINT('',#24586);
#6524=VERTEX_POINT('',#24597);
#6525=VERTEX_POINT('',#24607);
#6526=VERTEX_POINT('',#24608);
#6527=VERTEX_POINT('',#24655);
#6528=VERTEX_POINT('',#24656);
#6529=VERTEX_POINT('',#24703);
#6530=VERTEX_POINT('',#24704);
#6531=VERTEX_POINT('',#24757);
#6532=VERTEX_POINT('',#24758);
#6533=VERTEX_POINT('',#24805);
#6534=VERTEX_POINT('',#24806);
#6535=VERTEX_POINT('',#24853);
#6536=VERTEX_POINT('',#24854);
#6537=VERTEX_POINT('',#24856);
#6538=VERTEX_POINT('',#24864);
#6539=VERTEX_POINT('',#24872);
#6540=VERTEX_POINT('',#24873);
#6541=VERTEX_POINT('',#24897);
#6542=VERTEX_POINT('',#24898);
#6543=VERTEX_POINT('',#24921);
#6544=VERTEX_POINT('',#24922);
#6545=VERTEX_POINT('',#24946);
#6546=VERTEX_POINT('',#24947);
#6547=VERTEX_POINT('',#24971);
#6548=VERTEX_POINT('',#24972);
#6549=VERTEX_POINT('',#24995);
#6550=VERTEX_POINT('',#25048);
#6551=VERTEX_POINT('',#25050);
#6552=VERTEX_POINT('',#25305);
#6553=VERTEX_POINT('',#25368);
#6554=VERTEX_POINT('',#25371);
#6555=VERTEX_POINT('',#25633);
#6556=VERTEX_POINT('',#25634);
#6557=VERTEX_POINT('',#25638);
#6558=VERTEX_POINT('',#25642);
#6559=VERTEX_POINT('',#25646);
#6560=VERTEX_POINT('',#25650);
#6561=VERTEX_POINT('',#25657);
#6562=VERTEX_POINT('',#25658);
#6563=VERTEX_POINT('',#25660);
#6564=VERTEX_POINT('',#25665);
#6565=VERTEX_POINT('',#25669);
#6566=VERTEX_POINT('',#25674);
#6567=VERTEX_POINT('',#25678);
#6568=VERTEX_POINT('',#25683);
#6569=VERTEX_POINT('',#25687);
#6570=VERTEX_POINT('',#25692);
#6571=VERTEX_POINT('',#25696);
#6572=VERTEX_POINT('',#25701);
#6573=VERTEX_POINT('',#25705);
#6574=VERTEX_POINT('',#25710);
#6575=VERTEX_POINT('',#25716);
#6576=VERTEX_POINT('',#25718);
#6577=VERTEX_POINT('',#25722);
#6578=VERTEX_POINT('',#25726);
#6579=VERTEX_POINT('',#25730);
#6580=VERTEX_POINT('',#25734);
#6581=VERTEX_POINT('',#25738);
#6582=VERTEX_POINT('',#25742);
#6583=VERTEX_POINT('',#25746);
#6584=VERTEX_POINT('',#25750);
#6585=VERTEX_POINT('',#25761);
#6586=VERTEX_POINT('',#25769);
#6587=VERTEX_POINT('',#25782);
#6588=VERTEX_POINT('',#25789);
#8298=EDGE_CURVE('',#6521,#6522,#4111,.T.);
#8299=EDGE_CURVE('',#6521,#6523,#560,.T.);
#8300=EDGE_CURVE('',#6523,#6524,#1363,.T.);
#8301=EDGE_CURVE('',#6524,#6522,#561,.T.);
#8302=EDGE_CURVE('',#6525,#6526,#4112,.T.);
#8303=EDGE_CURVE('',#6525,#6521,#562,.T.);
#8304=EDGE_CURVE('',#6522,#6526,#563,.T.);
#8305=EDGE_CURVE('',#6527,#6528,#4113,.T.);
#8306=EDGE_CURVE('',#6527,#6525,#564,.T.);
#8307=EDGE_CURVE('',#6526,#6528,#565,.T.);
#8308=EDGE_CURVE('',#6529,#6530,#4114,.T.);
#8309=EDGE_CURVE('',#6529,#6527,#566,.T.);
#8310=EDGE_CURVE('',#6528,#6530,#567,.T.);
#8311=EDGE_CURVE('',#6531,#6532,#4115,.T.);
#8312=EDGE_CURVE('',#6531,#6529,#568,.T.);
#8313=EDGE_CURVE('',#6530,#6532,#569,.T.);
#8314=EDGE_CURVE('',#6533,#6534,#4116,.T.);
#8315=EDGE_CURVE('',#6533,#6531,#570,.T.);
#8316=EDGE_CURVE('',#6532,#6534,#571,.T.);
#8317=EDGE_CURVE('',#6535,#6536,#4117,.T.);
#8318=EDGE_CURVE('',#6535,#6537,#572,.T.);
#8319=EDGE_CURVE('',#6538,#6537,#1364,.T.);
#8320=EDGE_CURVE('',#6536,#6538,#573,.T.);
#8321=EDGE_CURVE('',#6539,#6540,#4118,.T.);
#8322=EDGE_CURVE('',#6539,#6535,#574,.T.);
#8323=EDGE_CURVE('',#6540,#6536,#575,.T.);
#8324=EDGE_CURVE('',#6541,#6542,#4119,.T.);
#8325=EDGE_CURVE('',#6541,#6539,#576,.T.);
#8326=EDGE_CURVE('',#6542,#6540,#577,.T.);
#8327=EDGE_CURVE('',#6543,#6544,#4120,.T.);
#8328=EDGE_CURVE('',#6543,#6541,#578,.T.);
#8329=EDGE_CURVE('',#6544,#6542,#579,.T.);
#8330=EDGE_CURVE('',#6545,#6546,#4121,.T.);
#8331=EDGE_CURVE('',#6545,#6543,#580,.T.);
#8332=EDGE_CURVE('',#6546,#6544,#581,.T.);
#8333=EDGE_CURVE('',#6547,#6548,#4122,.T.);
#8334=EDGE_CURVE('',#6547,#6545,#582,.T.);
#8335=EDGE_CURVE('',#6548,#6546,#583,.T.);
#8336=EDGE_CURVE('',#6537,#6549,#584,.T.);
#8337=EDGE_CURVE('',#6550,#6549,#1365,.F.);
#8338=EDGE_CURVE('',#6551,#6550,#1366,.F.);
#8339=EDGE_CURVE('',#6551,#6538,#585,.T.);
#8340=EDGE_CURVE('',#6534,#6551,#586,.T.);
#8341=EDGE_CURVE('',#6552,#6524,#587,.T.);
#8342=EDGE_CURVE('',#6552,#6548,#588,.T.);
#8343=EDGE_CURVE('',#6524,#6553,#1367,.T.);
#8344=EDGE_CURVE('',#6553,#6523,#1368,.T.);
#8345=EDGE_CURVE('',#6523,#6554,#589,.T.);
#8346=EDGE_CURVE('',#6554,#6552,#1369,.T.);
#8347=EDGE_CURVE('',#6554,#6547,#590,.T.);
#8348=EDGE_CURVE('',#6549,#6533,#591,.T.);
#8349=EDGE_CURVE('',#6555,#6556,#4123,.T.);
#8350=EDGE_CURVE('',#6556,#6555,#1370,.T.);
#8351=EDGE_CURVE('',#6556,#6557,#4124,.T.);
#8352=EDGE_CURVE('',#6557,#6556,#1371,.T.);
#8353=EDGE_CURVE('',#6557,#6558,#4125,.T.);
#8354=EDGE_CURVE('',#6558,#6557,#1372,.T.);
#8355=EDGE_CURVE('',#6558,#6559,#4126,.T.);
#8356=EDGE_CURVE('',#6559,#6558,#1373,.T.);
#8357=EDGE_CURVE('',#6559,#6560,#4127,.T.);
#8358=EDGE_CURVE('',#6560,#6559,#1374,.T.);
#8359=EDGE_CURVE('',#6560,#6555,#4128,.T.);
#8360=EDGE_CURVE('',#6555,#6560,#1375,.T.);
#8361=EDGE_CURVE('',#6561,#6562,#4129,.T.);
#8362=EDGE_CURVE('',#6563,#6562,#1376,.T.);
#8363=EDGE_CURVE('',#6557,#6563,#106,.T.);
#8364=EDGE_CURVE('',#6564,#6556,#107,.T.);
#8365=EDGE_CURVE('',#6565,#6564,#1377,.T.);
#8366=EDGE_CURVE('',#6556,#6565,#108,.T.);
#8367=EDGE_CURVE('',#6566,#6555,#109,.T.);
#8368=EDGE_CURVE('',#6567,#6566,#1378,.T.);
#8369=EDGE_CURVE('',#6555,#6567,#110,.T.);
#8370=EDGE_CURVE('',#6568,#6560,#111,.T.);
#8371=EDGE_CURVE('',#6569,#6568,#1379,.T.);
#8372=EDGE_CURVE('',#6560,#6569,#112,.T.);
#8373=EDGE_CURVE('',#6570,#6559,#113,.T.);
#8374=EDGE_CURVE('',#6571,#6570,#1380,.T.);
#8375=EDGE_CURVE('',#6559,#6571,#114,.T.);
#8376=EDGE_CURVE('',#6572,#6558,#115,.T.);
#8377=EDGE_CURVE('',#6573,#6572,#1381,.T.);
#8378=EDGE_CURVE('',#6558,#6573,#116,.T.);
#8379=EDGE_CURVE('',#6574,#6557,#117,.T.);
#8380=EDGE_CURVE('',#6562,#6574,#1382,.T.);
#8381=EDGE_CURVE('',#6575,#6558,#4130,.T.);
#8382=EDGE_CURVE('',#6576,#6575,#4131,.T.);
#8383=EDGE_CURVE('',#6576,#6557,#4132,.T.);
#8384=EDGE_CURVE('',#6557,#6577,#4133,.T.);
#8385=EDGE_CURVE('',#6577,#6574,#4134,.T.);
#8386=EDGE_CURVE('',#6578,#6559,#4135,.T.);
#8387=EDGE_CURVE('',#6575,#6578,#4136,.T.);
#8388=EDGE_CURVE('',#6571,#6579,#4137,.T.);
#8389=EDGE_CURVE('',#6559,#6579,#4138,.T.);
#8390=EDGE_CURVE('',#6558,#6580,#4139,.T.);
#8391=EDGE_CURVE('',#6580,#6572,#4140,.T.);
#8392=EDGE_CURVE('',#6581,#6576,#4141,.T.);
#8393=EDGE_CURVE('',#6581,#6556,#4142,.T.);
#8394=EDGE_CURVE('',#6556,#6582,#4143,.T.);
#8395=EDGE_CURVE('',#6582,#6564,#4144,.T.);
#8396=EDGE_CURVE('',#6583,#6560,#4145,.T.);
#8397=EDGE_CURVE('',#6578,#6583,#4146,.T.);
#8398=EDGE_CURVE('',#6569,#6584,#4147,.T.);
#8399=EDGE_CURVE('',#6560,#6584,#4148,.T.);
#8400=EDGE_CURVE('',#6579,#6570,#4149,.T.);
#8401=EDGE_CURVE('',#6573,#6580,#4150,.T.);
#8402=EDGE_CURVE('',#6584,#6568,#4151,.T.);
#8403=EDGE_CURVE('',#6585,#6566,#4152,.T.);
#8404=EDGE_CURVE('',#6567,#6585,#4153,.T.);
#8405=EDGE_CURVE('',#6565,#6582,#4154,.T.);
#8406=EDGE_CURVE('',#6563,#6577,#4155,.T.);
#8407=EDGE_CURVE('',#6586,#6555,#4156,.T.);
#8408=EDGE_CURVE('',#6583,#6586,#4157,.T.);
#8409=EDGE_CURVE('',#6555,#6585,#4158,.T.);
#8410=EDGE_CURVE('',#6586,#6581,#4159,.T.);
#8411=EDGE_CURVE('',#6587,#6587,#1383,.T.);
#8412=EDGE_CURVE('',#6553,#6587,#4160,.T.);
#8413=EDGE_CURVE('',#6549,#6551,#1384,.F.);
#8414=EDGE_CURVE('',#6588,#6588,#1385,.T.);
#8415=EDGE_CURVE('',#6588,#6550,#4161,.T.);
#11365=ORIENTED_EDGE('',*,*,#8298,.F.);
#11366=ORIENTED_EDGE('',*,*,#8299,.T.);
#11367=ORIENTED_EDGE('',*,*,#8300,.T.);
#11368=ORIENTED_EDGE('',*,*,#8301,.T.);
#11369=ORIENTED_EDGE('',*,*,#8302,.F.);
#11370=ORIENTED_EDGE('',*,*,#8303,.T.);
#11371=ORIENTED_EDGE('',*,*,#8298,.T.);
#11372=ORIENTED_EDGE('',*,*,#8304,.T.);
#11373=ORIENTED_EDGE('',*,*,#8305,.F.);
#11374=ORIENTED_EDGE('',*,*,#8306,.T.);
#11375=ORIENTED_EDGE('',*,*,#8302,.T.);
#11376=ORIENTED_EDGE('',*,*,#8307,.T.);
#11377=ORIENTED_EDGE('',*,*,#8308,.F.);
#11378=ORIENTED_EDGE('',*,*,#8309,.T.);
#11379=ORIENTED_EDGE('',*,*,#8305,.T.);
#11380=ORIENTED_EDGE('',*,*,#8310,.T.);
#11381=ORIENTED_EDGE('',*,*,#8311,.F.);
#11382=ORIENTED_EDGE('',*,*,#8312,.T.);
#11383=ORIENTED_EDGE('',*,*,#8308,.T.);
#11384=ORIENTED_EDGE('',*,*,#8313,.T.);
#11385=ORIENTED_EDGE('',*,*,#8314,.F.);
#11386=ORIENTED_EDGE('',*,*,#8315,.T.);
#11387=ORIENTED_EDGE('',*,*,#8311,.T.);
#11388=ORIENTED_EDGE('',*,*,#8316,.T.);
#11389=ORIENTED_EDGE('',*,*,#8317,.F.);
#11390=ORIENTED_EDGE('',*,*,#8318,.T.);
#11391=ORIENTED_EDGE('',*,*,#8319,.F.);
#11392=ORIENTED_EDGE('',*,*,#8320,.F.);
#11393=ORIENTED_EDGE('',*,*,#8321,.F.);
#11394=ORIENTED_EDGE('',*,*,#8322,.T.);
#11395=ORIENTED_EDGE('',*,*,#8317,.T.);
#11396=ORIENTED_EDGE('',*,*,#8323,.F.);
#11397=ORIENTED_EDGE('',*,*,#8324,.F.);
#11398=ORIENTED_EDGE('',*,*,#8325,.T.);
#11399=ORIENTED_EDGE('',*,*,#8321,.T.);
#11400=ORIENTED_EDGE('',*,*,#8326,.F.);
#11401=ORIENTED_EDGE('',*,*,#8327,.F.);
#11402=ORIENTED_EDGE('',*,*,#8328,.T.);
#11403=ORIENTED_EDGE('',*,*,#8324,.T.);
#11404=ORIENTED_EDGE('',*,*,#8329,.F.);
#11405=ORIENTED_EDGE('',*,*,#8330,.F.);
#11406=ORIENTED_EDGE('',*,*,#8331,.T.);
#11407=ORIENTED_EDGE('',*,*,#8327,.T.);
#11408=ORIENTED_EDGE('',*,*,#8332,.F.);
#11409=ORIENTED_EDGE('',*,*,#8333,.F.);
#11410=ORIENTED_EDGE('',*,*,#8334,.T.);
#11411=ORIENTED_EDGE('',*,*,#8330,.T.);
#11412=ORIENTED_EDGE('',*,*,#8335,.F.);
#11413=ORIENTED_EDGE('',*,*,#8319,.T.);
#11414=ORIENTED_EDGE('',*,*,#8336,.T.);
#11415=ORIENTED_EDGE('',*,*,#8337,.F.);
#11416=ORIENTED_EDGE('',*,*,#8338,.F.);
#11417=ORIENTED_EDGE('',*,*,#8339,.T.);
#11418=ORIENTED_EDGE('',*,*,#8339,.F.);
#11419=ORIENTED_EDGE('',*,*,#8340,.F.);
#11420=ORIENTED_EDGE('',*,*,#8316,.F.);
#11421=ORIENTED_EDGE('',*,*,#8313,.F.);
#11422=ORIENTED_EDGE('',*,*,#8310,.F.);
#11423=ORIENTED_EDGE('',*,*,#8307,.F.);
#11424=ORIENTED_EDGE('',*,*,#8304,.F.);
#11425=ORIENTED_EDGE('',*,*,#8301,.F.);
#11426=ORIENTED_EDGE('',*,*,#8341,.F.);
#11427=ORIENTED_EDGE('',*,*,#8342,.T.);
#11428=ORIENTED_EDGE('',*,*,#8335,.T.);
#11429=ORIENTED_EDGE('',*,*,#8332,.T.);
#11430=ORIENTED_EDGE('',*,*,#8329,.T.);
#11431=ORIENTED_EDGE('',*,*,#8326,.T.);
#11432=ORIENTED_EDGE('',*,*,#8323,.T.);
#11433=ORIENTED_EDGE('',*,*,#8320,.T.);
#11434=ORIENTED_EDGE('',*,*,#8343,.T.);
#11435=ORIENTED_EDGE('',*,*,#8344,.T.);
#11436=ORIENTED_EDGE('',*,*,#8345,.T.);
#11437=ORIENTED_EDGE('',*,*,#8346,.T.);
#11438=ORIENTED_EDGE('',*,*,#8341,.T.);
#11439=ORIENTED_EDGE('',*,*,#8333,.T.);
#11440=ORIENTED_EDGE('',*,*,#8342,.F.);
#11441=ORIENTED_EDGE('',*,*,#8346,.F.);
#11442=ORIENTED_EDGE('',*,*,#8347,.T.);
#11443=ORIENTED_EDGE('',*,*,#8336,.F.);
#11444=ORIENTED_EDGE('',*,*,#8318,.F.);
#11445=ORIENTED_EDGE('',*,*,#8322,.F.);
#11446=ORIENTED_EDGE('',*,*,#8325,.F.);
#11447=ORIENTED_EDGE('',*,*,#8328,.F.);
#11448=ORIENTED_EDGE('',*,*,#8331,.F.);
#11449=ORIENTED_EDGE('',*,*,#8334,.F.);
#11450=ORIENTED_EDGE('',*,*,#8347,.F.);
#11451=ORIENTED_EDGE('',*,*,#8345,.F.);
#11452=ORIENTED_EDGE('',*,*,#8299,.F.);
#11453=ORIENTED_EDGE('',*,*,#8303,.F.);
#11454=ORIENTED_EDGE('',*,*,#8306,.F.);
#11455=ORIENTED_EDGE('',*,*,#8309,.F.);
#11456=ORIENTED_EDGE('',*,*,#8312,.F.);
#11457=ORIENTED_EDGE('',*,*,#8315,.F.);
#11458=ORIENTED_EDGE('',*,*,#8348,.F.);
#11459=ORIENTED_EDGE('',*,*,#8349,.F.);
#11460=ORIENTED_EDGE('',*,*,#8350,.F.);
#11461=ORIENTED_EDGE('',*,*,#8351,.F.);
#11462=ORIENTED_EDGE('',*,*,#8352,.F.);
#11463=ORIENTED_EDGE('',*,*,#8353,.F.);
#11464=ORIENTED_EDGE('',*,*,#8354,.F.);
#11465=ORIENTED_EDGE('',*,*,#8355,.F.);
#11466=ORIENTED_EDGE('',*,*,#8356,.F.);
#11467=ORIENTED_EDGE('',*,*,#8357,.F.);
#11468=ORIENTED_EDGE('',*,*,#8358,.F.);
#11469=ORIENTED_EDGE('',*,*,#8359,.F.);
#11470=ORIENTED_EDGE('',*,*,#8360,.F.);
#11471=ORIENTED_EDGE('',*,*,#8361,.T.);
#11472=ORIENTED_EDGE('',*,*,#8362,.F.);
#11473=ORIENTED_EDGE('',*,*,#8363,.F.);
#11474=ORIENTED_EDGE('',*,*,#8352,.T.);
#11475=ORIENTED_EDGE('',*,*,#8364,.F.);
#11476=ORIENTED_EDGE('',*,*,#8365,.F.);
#11477=ORIENTED_EDGE('',*,*,#8366,.F.);
#11478=ORIENTED_EDGE('',*,*,#8350,.T.);
#11479=ORIENTED_EDGE('',*,*,#8367,.F.);
#11480=ORIENTED_EDGE('',*,*,#8368,.F.);
#11481=ORIENTED_EDGE('',*,*,#8369,.F.);
#11482=ORIENTED_EDGE('',*,*,#8360,.T.);
#11483=ORIENTED_EDGE('',*,*,#8370,.F.);
#11484=ORIENTED_EDGE('',*,*,#8371,.F.);
#11485=ORIENTED_EDGE('',*,*,#8372,.F.);
#11486=ORIENTED_EDGE('',*,*,#8358,.T.);
#11487=ORIENTED_EDGE('',*,*,#8373,.F.);
#11488=ORIENTED_EDGE('',*,*,#8374,.F.);
#11489=ORIENTED_EDGE('',*,*,#8375,.F.);
#11490=ORIENTED_EDGE('',*,*,#8356,.T.);
#11491=ORIENTED_EDGE('',*,*,#8376,.F.);
#11492=ORIENTED_EDGE('',*,*,#8377,.F.);
#11493=ORIENTED_EDGE('',*,*,#8378,.F.);
#11494=ORIENTED_EDGE('',*,*,#8354,.T.);
#11495=ORIENTED_EDGE('',*,*,#8379,.F.);
#11496=ORIENTED_EDGE('',*,*,#8380,.F.);
#11497=ORIENTED_EDGE('',*,*,#8361,.F.);
#11498=ORIENTED_EDGE('',*,*,#8353,.T.);
#11499=ORIENTED_EDGE('',*,*,#8381,.F.);
#11500=ORIENTED_EDGE('',*,*,#8382,.F.);
#11501=ORIENTED_EDGE('',*,*,#8383,.T.);
#11502=ORIENTED_EDGE('',*,*,#8379,.T.);
#11503=ORIENTED_EDGE('',*,*,#8384,.T.);
#11504=ORIENTED_EDGE('',*,*,#8385,.T.);
#11505=ORIENTED_EDGE('',*,*,#8355,.T.);
#11506=ORIENTED_EDGE('',*,*,#8386,.F.);
#11507=ORIENTED_EDGE('',*,*,#8387,.F.);
#11508=ORIENTED_EDGE('',*,*,#8381,.T.);
#11509=ORIENTED_EDGE('',*,*,#8375,.T.);
#11510=ORIENTED_EDGE('',*,*,#8388,.T.);
#11511=ORIENTED_EDGE('',*,*,#8389,.F.);
#11512=ORIENTED_EDGE('',*,*,#8376,.T.);
#11513=ORIENTED_EDGE('',*,*,#8390,.T.);
#11514=ORIENTED_EDGE('',*,*,#8391,.T.);
#11515=ORIENTED_EDGE('',*,*,#8351,.T.);
#11516=ORIENTED_EDGE('',*,*,#8383,.F.);
#11517=ORIENTED_EDGE('',*,*,#8392,.F.);
#11518=ORIENTED_EDGE('',*,*,#8393,.T.);
#11519=ORIENTED_EDGE('',*,*,#8364,.T.);
#11520=ORIENTED_EDGE('',*,*,#8394,.T.);
#11521=ORIENTED_EDGE('',*,*,#8395,.T.);
#11522=ORIENTED_EDGE('',*,*,#8357,.T.);
#11523=ORIENTED_EDGE('',*,*,#8396,.F.);
#11524=ORIENTED_EDGE('',*,*,#8397,.F.);
#11525=ORIENTED_EDGE('',*,*,#8386,.T.);
#11526=ORIENTED_EDGE('',*,*,#8372,.T.);
#11527=ORIENTED_EDGE('',*,*,#8398,.T.);
#11528=ORIENTED_EDGE('',*,*,#8399,.F.);
#11529=ORIENTED_EDGE('',*,*,#8373,.T.);
#11530=ORIENTED_EDGE('',*,*,#8389,.T.);
#11531=ORIENTED_EDGE('',*,*,#8400,.T.);
#11532=ORIENTED_EDGE('',*,*,#8377,.T.);
#11533=ORIENTED_EDGE('',*,*,#8391,.F.);
#11534=ORIENTED_EDGE('',*,*,#8401,.F.);
#11535=ORIENTED_EDGE('',*,*,#8374,.T.);
#11536=ORIENTED_EDGE('',*,*,#8400,.F.);
#11537=ORIENTED_EDGE('',*,*,#8388,.F.);
#11538=ORIENTED_EDGE('',*,*,#8371,.T.);
#11539=ORIENTED_EDGE('',*,*,#8402,.F.);
#11540=ORIENTED_EDGE('',*,*,#8398,.F.);
#11541=ORIENTED_EDGE('',*,*,#8368,.T.);
#11542=ORIENTED_EDGE('',*,*,#8403,.F.);
#11543=ORIENTED_EDGE('',*,*,#8404,.F.);
#11544=ORIENTED_EDGE('',*,*,#8365,.T.);
#11545=ORIENTED_EDGE('',*,*,#8395,.F.);
#11546=ORIENTED_EDGE('',*,*,#8405,.F.);
#11547=ORIENTED_EDGE('',*,*,#8362,.T.);
#11548=ORIENTED_EDGE('',*,*,#8380,.T.);
#11549=ORIENTED_EDGE('',*,*,#8385,.F.);
#11550=ORIENTED_EDGE('',*,*,#8406,.F.);
#11551=ORIENTED_EDGE('',*,*,#8359,.T.);
#11552=ORIENTED_EDGE('',*,*,#8407,.F.);
#11553=ORIENTED_EDGE('',*,*,#8408,.F.);
#11554=ORIENTED_EDGE('',*,*,#8396,.T.);
#11555=ORIENTED_EDGE('',*,*,#8369,.T.);
#11556=ORIENTED_EDGE('',*,*,#8404,.T.);
#11557=ORIENTED_EDGE('',*,*,#8409,.F.);
#11558=ORIENTED_EDGE('',*,*,#8370,.T.);
#11559=ORIENTED_EDGE('',*,*,#8399,.T.);
#11560=ORIENTED_EDGE('',*,*,#8402,.T.);
#11561=ORIENTED_EDGE('',*,*,#8367,.T.);
#11562=ORIENTED_EDGE('',*,*,#8409,.T.);
#11563=ORIENTED_EDGE('',*,*,#8403,.T.);
#11564=ORIENTED_EDGE('',*,*,#8349,.T.);
#11565=ORIENTED_EDGE('',*,*,#8393,.F.);
#11566=ORIENTED_EDGE('',*,*,#8410,.F.);
#11567=ORIENTED_EDGE('',*,*,#8407,.T.);
#11568=ORIENTED_EDGE('',*,*,#8378,.T.);
#11569=ORIENTED_EDGE('',*,*,#8401,.T.);
#11570=ORIENTED_EDGE('',*,*,#8390,.F.);
#11571=ORIENTED_EDGE('',*,*,#8363,.T.);
#11572=ORIENTED_EDGE('',*,*,#8406,.T.);
#11573=ORIENTED_EDGE('',*,*,#8384,.F.);
#11574=ORIENTED_EDGE('',*,*,#8366,.T.);
#11575=ORIENTED_EDGE('',*,*,#8405,.T.);
#11576=ORIENTED_EDGE('',*,*,#8394,.F.);
#11577=ORIENTED_EDGE('',*,*,#8411,.F.);
#11578=ORIENTED_EDGE('',*,*,#8343,.F.);
#11579=ORIENTED_EDGE('',*,*,#8300,.F.);
#11580=ORIENTED_EDGE('',*,*,#8344,.F.);
#11581=ORIENTED_EDGE('',*,*,#8412,.T.);
#11582=ORIENTED_EDGE('',*,*,#8411,.T.);
#11583=ORIENTED_EDGE('',*,*,#8412,.F.);
#11584=ORIENTED_EDGE('',*,*,#8314,.T.);
#11585=ORIENTED_EDGE('',*,*,#8340,.T.);
#11586=ORIENTED_EDGE('',*,*,#8413,.F.);
#11587=ORIENTED_EDGE('',*,*,#8348,.T.);
#11588=ORIENTED_EDGE('',*,*,#8414,.F.);
#11589=ORIENTED_EDGE('',*,*,#8415,.T.);
#11590=ORIENTED_EDGE('',*,*,#8337,.T.);
#11591=ORIENTED_EDGE('',*,*,#8413,.T.);
#11592=ORIENTED_EDGE('',*,*,#8338,.T.);
#11593=ORIENTED_EDGE('',*,*,#8415,.F.);
#11594=ORIENTED_EDGE('',*,*,#8414,.T.);
#11595=ORIENTED_EDGE('',*,*,#8397,.T.);
#11596=ORIENTED_EDGE('',*,*,#8408,.T.);
#11597=ORIENTED_EDGE('',*,*,#8410,.T.);
#11598=ORIENTED_EDGE('',*,*,#8392,.T.);
#11599=ORIENTED_EDGE('',*,*,#8382,.T.);
#11600=ORIENTED_EDGE('',*,*,#8387,.T.);
#14965=PLANE('',#16849);
#14966=PLANE('',#16852);
#14967=PLANE('',#16857);
#14968=PLANE('',#16859);
#14969=PLANE('',#16861);
#14970=PLANE('',#16863);
#14971=PLANE('',#16865);
#14972=PLANE('',#16867);
#14973=PLANE('',#16877);
#14974=PLANE('',#16878);
#14975=PLANE('',#16879);
#14976=PLANE('',#16880);
#14977=PLANE('',#16881);
#14978=PLANE('',#16882);
#14979=PLANE('',#16883);
#14980=PLANE('',#16884);
#14981=PLANE('',#16885);
#14982=PLANE('',#16886);
#14983=PLANE('',#16887);
#14984=PLANE('',#16888);
#14985=PLANE('',#16889);
#14986=PLANE('',#16890);
#14987=PLANE('',#16891);
#14988=PLANE('',#16892);
#14989=PLANE('',#16893);
#14990=PLANE('',#16894);
#14991=PLANE('',#16895);
#14992=PLANE('',#16896);
#14993=PLANE('',#16897);
#14994=PLANE('',#16898);
#14995=PLANE('',#16899);
#14996=PLANE('',#16900);
#14997=PLANE('',#16901);
#14998=PLANE('',#16908);
#15590=ADVANCED_FACE('',(#2047),#916,.T.);
#15591=ADVANCED_FACE('',(#2048),#917,.T.);
#15592=ADVANCED_FACE('',(#2049),#918,.T.);
#15593=ADVANCED_FACE('',(#2050),#919,.T.);
#15594=ADVANCED_FACE('',(#2051),#920,.T.);
#15595=ADVANCED_FACE('',(#2052),#921,.T.);
#15596=ADVANCED_FACE('',(#2053),#922,.T.);
#15597=ADVANCED_FACE('',(#2054),#923,.T.);
#15598=ADVANCED_FACE('',(#2055),#924,.T.);
#15599=ADVANCED_FACE('',(#2056),#925,.T.);
#15600=ADVANCED_FACE('',(#2057),#926,.T.);
#15601=ADVANCED_FACE('',(#2058),#927,.T.);
#15602=ADVANCED_FACE('',(#2059),#14965,.F.);
#15603=ADVANCED_FACE('',(#2060),#497,.F.);
#15604=ADVANCED_FACE('',(#2061),#14966,.T.);
#15605=ADVANCED_FACE('',(#2062),#928,.T.);
#15606=ADVANCED_FACE('',(#2063),#498,.F.);
#15607=ADVANCED_FACE('',(#2064),#14967,.F.);
#15608=ADVANCED_FACE('',(#2065),#14968,.F.);
#15609=ADVANCED_FACE('',(#2066),#14969,.F.);
#15610=ADVANCED_FACE('',(#2067),#14970,.F.);
#15611=ADVANCED_FACE('',(#2068),#14971,.F.);
#15612=ADVANCED_FACE('',(#2069),#14972,.F.);
#15613=ADVANCED_FACE('',(#2070),#1740,.F.);
#15614=ADVANCED_FACE('',(#2071),#14973,.F.);
#15615=ADVANCED_FACE('',(#2072),#14974,.F.);
#15616=ADVANCED_FACE('',(#2073),#14975,.F.);
#15617=ADVANCED_FACE('',(#2074),#14976,.F.);
#15618=ADVANCED_FACE('',(#2075),#14977,.F.);
#15619=ADVANCED_FACE('',(#2076),#14978,.F.);
#15620=ADVANCED_FACE('',(#2077),#14979,.F.);
#15621=ADVANCED_FACE('',(#2078),#14980,.F.);
#15622=ADVANCED_FACE('',(#2079),#14981,.F.);
#15623=ADVANCED_FACE('',(#2080),#14982,.F.);
#15624=ADVANCED_FACE('',(#2081),#14983,.F.);
#15625=ADVANCED_FACE('',(#2082),#14984,.F.);
#15626=ADVANCED_FACE('',(#2083),#14985,.F.);
#15627=ADVANCED_FACE('',(#2084),#14986,.F.);
#15628=ADVANCED_FACE('',(#2085),#14987,.F.);
#15629=ADVANCED_FACE('',(#2086),#14988,.F.);
#15630=ADVANCED_FACE('',(#2087),#14989,.F.);
#15631=ADVANCED_FACE('',(#2088),#14990,.F.);
#15632=ADVANCED_FACE('',(#2089),#14991,.F.);
#15633=ADVANCED_FACE('',(#2090),#14992,.F.);
#15634=ADVANCED_FACE('',(#2091),#14993,.F.);
#15635=ADVANCED_FACE('',(#2092),#14994,.F.);
#15636=ADVANCED_FACE('',(#2093),#14995,.F.);
#15637=ADVANCED_FACE('',(#2094),#14996,.F.);
#15638=ADVANCED_FACE('',(#2095),#14997,.T.);
#15639=ADVANCED_FACE('',(#2096),#1741,.T.);
#15640=ADVANCED_FACE('',(#2097),#929,.T.);
#15641=ADVANCED_FACE('',(#2098),#1742,.T.);
#15642=ADVANCED_FACE('',(#2099,#1186),#14998,.T.);
#16240=CLOSED_SHELL('',(#15590,#15591,#15592,#15593,#15594,#15595,#15596,
#15597,#15598,#15599,#15600,#15601,#15602,#15603,#15604,#15605,#15606,#15607,
#15608,#15609,#15610,#15611,#15612,#15613,#15614,#15615,#15616,#15617,#15618,
#15619,#15620,#15621,#15622,#15623,#15624,#15625,#15626,#15627,#15628,#15629,
#15630,#15631,#15632,#15633,#15634,#15635,#15636,#15637,#15638,#15639,#15640,
#15641,#15642));
#16834=AXIS2_PLACEMENT_3D('',#24581,#19124,#19125);
#16835=AXIS2_PLACEMENT_3D('',#24582,#19126,#19127);
#16836=AXIS2_PLACEMENT_3D('',#24598,#19129,#19130);
#16837=AXIS2_PLACEMENT_3D('',#24606,#19131,#19132);
#16838=AXIS2_PLACEMENT_3D('',#24654,#19134,#19135);
#16839=AXIS2_PLACEMENT_3D('',#24702,#19137,#19138);
#16840=AXIS2_PLACEMENT_3D('',#24756,#19140,#19141);
#16841=AXIS2_PLACEMENT_3D('',#24804,#19143,#19144);
#16842=AXIS2_PLACEMENT_3D('',#24852,#19146,#19147);
#16843=AXIS2_PLACEMENT_3D('',#24865,#19149,#19150);
#16844=AXIS2_PLACEMENT_3D('',#24871,#19151,#19152);
#16845=AXIS2_PLACEMENT_3D('',#24896,#19154,#19155);
#16846=AXIS2_PLACEMENT_3D('',#24920,#19157,#19158);
#16847=AXIS2_PLACEMENT_3D('',#24945,#19160,#19161);
#16848=AXIS2_PLACEMENT_3D('',#24970,#19163,#19164);
#16849=AXIS2_PLACEMENT_3D('',#24994,#19166,#19167);
#16850=AXIS2_PLACEMENT_3D('',#25049,#19168,#19169);
#16851=AXIS2_PLACEMENT_3D('',#25051,#19170,#19171);
#16852=AXIS2_PLACEMENT_3D('',#25367,#19172,#19173);
#16853=AXIS2_PLACEMENT_3D('',#25369,#19174,#19175);
#16854=AXIS2_PLACEMENT_3D('',#25370,#19176,#19177);
#16855=AXIS2_PLACEMENT_3D('',#25427,#19178,#19179);
#16856=AXIS2_PLACEMENT_3D('',#25428,#19180,#19181);
#16857=AXIS2_PLACEMENT_3D('',#25632,#19182,#19183);
#16858=AXIS2_PLACEMENT_3D('',#25636,#19185,#19186);
#16859=AXIS2_PLACEMENT_3D('',#25637,#19187,#19188);
#16860=AXIS2_PLACEMENT_3D('',#25640,#19190,#19191);
#16861=AXIS2_PLACEMENT_3D('',#25641,#19192,#19193);
#16862=AXIS2_PLACEMENT_3D('',#25644,#19195,#19196);
#16863=AXIS2_PLACEMENT_3D('',#25645,#19197,#19198);
#16864=AXIS2_PLACEMENT_3D('',#25648,#19200,#19201);
#16865=AXIS2_PLACEMENT_3D('',#25649,#19202,#19203);
#16866=AXIS2_PLACEMENT_3D('',#25652,#19205,#19206);
#16867=AXIS2_PLACEMENT_3D('',#25653,#19207,#19208);
#16868=AXIS2_PLACEMENT_3D('',#25655,#19210,#19211);
#16869=AXIS2_PLACEMENT_3D('',#25656,#19212,#19213);
#16870=AXIS2_PLACEMENT_3D('',#25661,#19215,#19216);
#16871=AXIS2_PLACEMENT_3D('',#25670,#19217,#19218);
#16872=AXIS2_PLACEMENT_3D('',#25679,#19219,#19220);
#16873=AXIS2_PLACEMENT_3D('',#25688,#19221,#19222);
#16874=AXIS2_PLACEMENT_3D('',#25697,#19223,#19224);
#16875=AXIS2_PLACEMENT_3D('',#25706,#19225,#19226);
#16876=AXIS2_PLACEMENT_3D('',#25714,#19227,#19228);
#16877=AXIS2_PLACEMENT_3D('',#25715,#19229,#19230);
#16878=AXIS2_PLACEMENT_3D('',#25721,#19234,#19235);
#16879=AXIS2_PLACEMENT_3D('',#25725,#19238,#19239);
#16880=AXIS2_PLACEMENT_3D('',#25729,#19242,#19243);
#16881=AXIS2_PLACEMENT_3D('',#25733,#19246,#19247);
#16882=AXIS2_PLACEMENT_3D('',#25737,#19250,#19251);
#16883=AXIS2_PLACEMENT_3D('',#25741,#19254,#19255);
#16884=AXIS2_PLACEMENT_3D('',#25745,#19258,#19259);
#16885=AXIS2_PLACEMENT_3D('',#25749,#19262,#19263);
#16886=AXIS2_PLACEMENT_3D('',#25753,#19266,#19267);
#16887=AXIS2_PLACEMENT_3D('',#25755,#19269,#19270);
#16888=AXIS2_PLACEMENT_3D('',#25757,#19272,#19273);
#16889=AXIS2_PLACEMENT_3D('',#25758,#19274,#19275);
#16890=AXIS2_PLACEMENT_3D('',#25760,#19277,#19278);
#16891=AXIS2_PLACEMENT_3D('',#25764,#19281,#19282);
#16892=AXIS2_PLACEMENT_3D('',#25766,#19284,#19285);
#16893=AXIS2_PLACEMENT_3D('',#25768,#19287,#19288);
#16894=AXIS2_PLACEMENT_3D('',#25772,#19291,#19292);
#16895=AXIS2_PLACEMENT_3D('',#25774,#19294,#19295);
#16896=AXIS2_PLACEMENT_3D('',#25775,#19296,#19297);
#16897=AXIS2_PLACEMENT_3D('',#25776,#19298,#19299);
#16898=AXIS2_PLACEMENT_3D('',#25778,#19301,#19302);
#16899=AXIS2_PLACEMENT_3D('',#25779,#19303,#19304);
#16900=AXIS2_PLACEMENT_3D('',#25780,#19305,#19306);
#16901=AXIS2_PLACEMENT_3D('',#25781,#19307,#19308);
#16902=AXIS2_PLACEMENT_3D('',#25783,#19309,#19310);
#16903=AXIS2_PLACEMENT_3D('',#25784,#19311,#19312);
#16904=AXIS2_PLACEMENT_3D('',#25786,#19314,#19315);
#16905=AXIS2_PLACEMENT_3D('',#25787,#19316,#19317);
#16906=AXIS2_PLACEMENT_3D('',#25788,#19318,#19319);
#16907=AXIS2_PLACEMENT_3D('',#25790,#19320,#19321);
#16908=AXIS2_PLACEMENT_3D('',#25792,#19323,#19324);
#19124=DIRECTION('axis',(0.,0.,1.));
#19125=DIRECTION('refdir',(1.,0.,0.));
#19126=DIRECTION('center_axis',(0.,0.,1.));
#19127=DIRECTION('ref_axis',(1.,0.,0.));
#19128=DIRECTION('',(0.,0.,-1.));
#19129=DIRECTION('center_axis',(0.,0.,1.));
#19130=DIRECTION('ref_axis',(1.,0.,0.));
#19131=DIRECTION('center_axis',(0.,0.,1.));
#19132=DIRECTION('ref_axis',(1.,0.,0.));
#19133=DIRECTION('',(0.,0.,-1.));
#19134=DIRECTION('center_axis',(0.,0.,1.));
#19135=DIRECTION('ref_axis',(1.,0.,0.));
#19136=DIRECTION('',(0.,0.,-1.));
#19137=DIRECTION('center_axis',(0.,0.,1.));
#19138=DIRECTION('ref_axis',(1.,0.,0.));
#19139=DIRECTION('',(0.,0.,-1.));
#19140=DIRECTION('center_axis',(0.,0.,1.));
#19141=DIRECTION('ref_axis',(1.,0.,0.));
#19142=DIRECTION('',(0.,0.,-1.));
#19143=DIRECTION('center_axis',(0.,0.,1.));
#19144=DIRECTION('ref_axis',(1.,0.,0.));
#19145=DIRECTION('',(0.,0.,-1.));
#19146=DIRECTION('center_axis',(0.,0.,1.));
#19147=DIRECTION('ref_axis',(-0.131102582345095,-0.991368807711059,0.));
#19148=DIRECTION('',(0.,0.,1.));
#19149=DIRECTION('center_axis',(0.,0.,1.));
#19150=DIRECTION('ref_axis',(1.,1.81591784523378E-14,0.));
#19151=DIRECTION('center_axis',(0.,0.,1.));
#19152=DIRECTION('ref_axis',(1.,1.81591784523378E-14,0.));
#19153=DIRECTION('',(0.,0.,1.));
#19154=DIRECTION('center_axis',(0.,0.,1.));
#19155=DIRECTION('ref_axis',(1.,1.81591784523378E-14,0.));
#19156=DIRECTION('',(0.,0.,1.));
#19157=DIRECTION('center_axis',(0.,0.,1.));
#19158=DIRECTION('ref_axis',(1.,1.81591784523378E-14,0.));
#19159=DIRECTION('',(0.,0.,1.));
#19160=DIRECTION('center_axis',(0.,0.,1.));
#19161=DIRECTION('ref_axis',(1.,1.81591784523378E-14,0.));
#19162=DIRECTION('',(0.,0.,1.));
#19163=DIRECTION('center_axis',(0.,0.,1.));
#19164=DIRECTION('ref_axis',(1.,1.81591784523378E-14,0.));
#19165=DIRECTION('',(0.,0.,1.));
#19166=DIRECTION('center_axis',(0.,0.,1.));
#19167=DIRECTION('ref_axis',(1.,0.,0.));
#19168=DIRECTION('center_axis',(0.,0.,-1.));
#19169=DIRECTION('ref_axis',(1.,0.,0.));
#19170=DIRECTION('center_axis',(0.,0.,-1.));
#19171=DIRECTION('ref_axis',(1.,0.,0.));
#19172=DIRECTION('center_axis',(0.,0.,1.));
#19173=DIRECTION('ref_axis',(1.,0.,0.));
#19174=DIRECTION('center_axis',(0.,0.,1.));
#19175=DIRECTION('ref_axis',(1.,0.,0.));
#19176=DIRECTION('center_axis',(0.,0.,1.));
#19177=DIRECTION('ref_axis',(1.,0.,0.));
#19178=DIRECTION('center_axis',(0.,0.,-1.));
#19179=DIRECTION('ref_axis',(1.,1.81591784523378E-14,0.));
#19180=DIRECTION('center_axis',(0.,0.,1.));
#19181=DIRECTION('ref_axis',(1.,1.81591784523378E-14,0.));
#19182=DIRECTION('center_axis',(0.,0.,1.));
#19183=DIRECTION('ref_axis',(1.,0.,0.));
#19184=DIRECTION('',(-1.,2.40370335797945E-16,0.));
#19185=DIRECTION('center_axis',(0.,0.,1.));
#19186=DIRECTION('ref_axis',(1.,0.,0.));
#19187=DIRECTION('center_axis',(0.,0.,1.));
#19188=DIRECTION('ref_axis',(1.,0.,0.));
#19189=DIRECTION('',(-0.5,0.866025403784439,0.));
#19190=DIRECTION('center_axis',(0.,0.,1.));
#19191=DIRECTION('ref_axis',(1.,0.,0.));
#19192=DIRECTION('center_axis',(0.,0.,1.));
#19193=DIRECTION('ref_axis',(1.,0.,0.));
#19194=DIRECTION('',(0.5,0.866025403784439,0.));
#19195=DIRECTION('center_axis',(0.,0.,1.));
#19196=DIRECTION('ref_axis',(1.,0.,0.));
#19197=DIRECTION('center_axis',(0.,0.,1.));
#19198=DIRECTION('ref_axis',(1.,0.,0.));
#19199=DIRECTION('',(1.,-1.20185167898973E-16,0.));
#19200=DIRECTION('center_axis',(0.,0.,1.));
#19201=DIRECTION('ref_axis',(1.,0.,0.));
#19202=DIRECTION('center_axis',(0.,0.,1.));
#19203=DIRECTION('ref_axis',(1.,0.,0.));
#19204=DIRECTION('',(0.5,-0.866025403784439,0.));
#19205=DIRECTION('center_axis',(0.,0.,1.));
#19206=DIRECTION('ref_axis',(1.,0.,0.));
#19207=DIRECTION('center_axis',(0.,0.,1.));
#19208=DIRECTION('ref_axis',(1.,0.,0.));
#19209=DIRECTION('',(-0.5,-0.866025403784439,0.));
#19210=DIRECTION('center_axis',(0.,0.,1.));
#19211=DIRECTION('ref_axis',(1.,0.,0.));
#19212=DIRECTION('center_axis',(0.,0.,1.));
#19213=DIRECTION('ref_axis',(1.,0.,0.));
#19214=DIRECTION('',(-0.854211984955561,-1.04610797316913E-16,0.519924883765223));
#19215=DIRECTION('center_axis',(0.,0.,-1.));
#19216=DIRECTION('ref_axis',(1.,0.,0.));
#19217=DIRECTION('center_axis',(0.,0.,-1.));
#19218=DIRECTION('ref_axis',(1.,0.,0.));
#19219=DIRECTION('center_axis',(0.,0.,-1.));
#19220=DIRECTION('ref_axis',(1.,0.,0.));
#19221=DIRECTION('center_axis',(0.,0.,-1.));
#19222=DIRECTION('ref_axis',(1.,0.,0.));
#19223=DIRECTION('center_axis',(0.,0.,-1.));
#19224=DIRECTION('ref_axis',(1.,0.,0.));
#19225=DIRECTION('center_axis',(0.,0.,-1.));
#19226=DIRECTION('ref_axis',(1.,0.,0.));
#19227=DIRECTION('center_axis',(0.,0.,-1.));
#19228=DIRECTION('ref_axis',(1.,0.,0.));
#19229=DIRECTION('center_axis',(-0.866025403784439,0.5,0.));
#19230=DIRECTION('ref_axis',(0.5,0.866025403784439,0.));
#19231=DIRECTION('',(0.,0.,-1.));
#19232=DIRECTION('',(0.5,0.866025403784439,0.));
#19233=DIRECTION('',(0.,0.,-1.));
#19234=DIRECTION('center_axis',(-0.866025403784439,0.5,0.));
#19235=DIRECTION('ref_axis',(0.5,0.866025403784439,0.));
#19236=DIRECTION('',(0.,0.,-1.));
#19237=DIRECTION('',(0.5,0.866025403784439,0.));
#19238=DIRECTION('center_axis',(1.20185167898973E-16,1.,0.));
#19239=DIRECTION('ref_axis',(1.,-1.20185167898973E-16,0.));
#19240=DIRECTION('',(0.,0.,-1.));
#19241=DIRECTION('',(1.,-1.20185167898973E-16,0.));
#19242=DIRECTION('center_axis',(1.20185167898973E-16,1.,0.));
#19243=DIRECTION('ref_axis',(1.,-1.20185167898973E-16,0.));
#19244=DIRECTION('',(1.,-1.20185167898973E-16,0.));
#19245=DIRECTION('',(0.,0.,-1.));
#19246=DIRECTION('center_axis',(1.20185167898973E-16,1.,0.));
#19247=DIRECTION('ref_axis',(1.,-1.20185167898973E-16,0.));
#19248=DIRECTION('',(0.,0.,-1.));
#19249=DIRECTION('',(1.,-1.20185167898973E-16,0.));
#19250=DIRECTION('center_axis',(-0.866025403784439,-0.5,0.));
#19251=DIRECTION('ref_axis',(-0.5,0.866025403784439,0.));
#19252=DIRECTION('',(-0.5,0.866025403784439,0.));
#19253=DIRECTION('',(0.,0.,-1.));
#19254=DIRECTION('center_axis',(-0.866025403784439,-0.5,0.));
#19255=DIRECTION('ref_axis',(-0.5,0.866025403784439,0.));
#19256=DIRECTION('',(0.,0.,-1.));
#19257=DIRECTION('',(-0.5,0.866025403784439,0.));
#19258=DIRECTION('center_axis',(0.866025403784439,0.5,0.));
#19259=DIRECTION('ref_axis',(0.5,-0.866025403784439,0.));
#19260=DIRECTION('',(0.,0.,-1.));
#19261=DIRECTION('',(0.5,-0.866025403784439,0.));
#19262=DIRECTION('center_axis',(0.866025403784439,0.5,0.));
#19263=DIRECTION('ref_axis',(0.5,-0.866025403784439,0.));
#19264=DIRECTION('',(0.5,-0.866025403784439,0.));
#19265=DIRECTION('',(0.,0.,-1.));
#19266=DIRECTION('center_axis',(0.866025403784439,0.5,0.));
#19267=DIRECTION('ref_axis',(0.5,-0.866025403784439,0.));
#19268=DIRECTION('',(0.5,-0.866025403784439,0.));
#19269=DIRECTION('center_axis',(0.,0.,-1.));
#19270=DIRECTION('ref_axis',(-1.,0.,0.));
#19271=DIRECTION('',(0.5,0.866025403784439,0.));
#19272=DIRECTION('center_axis',(0.,0.,-1.));
#19273=DIRECTION('ref_axis',(-1.,0.,0.));
#19274=DIRECTION('center_axis',(0.,0.,-1.));
#19275=DIRECTION('ref_axis',(-1.,0.,0.));
#19276=DIRECTION('',(-0.5,-0.866025403784439,0.));
#19277=DIRECTION('center_axis',(0.,0.,-1.));
#19278=DIRECTION('ref_axis',(-1.,0.,0.));
#19279=DIRECTION('',(-1.,2.40370335797945E-16,0.));
#19280=DIRECTION('',(-0.5,-0.866025403784439,0.));
#19281=DIRECTION('center_axis',(0.,0.,-1.));
#19282=DIRECTION('ref_axis',(-1.,0.,0.));
#19283=DIRECTION('',(-1.,2.40370335797945E-16,0.));
#19284=DIRECTION('center_axis',(0.,0.,-1.));
#19285=DIRECTION('ref_axis',(-1.,0.,0.));
#19286=DIRECTION('',(-0.5,0.866025403784439,0.));
#19287=DIRECTION('center_axis',(0.866025403784439,-0.5,0.));
#19288=DIRECTION('ref_axis',(-0.5,-0.866025403784439,0.));
#19289=DIRECTION('',(0.,0.,-1.));
#19290=DIRECTION('',(-0.5,-0.866025403784439,0.));
#19291=DIRECTION('center_axis',(0.866025403784439,-0.5,0.));
#19292=DIRECTION('ref_axis',(-0.5,-0.866025403784439,0.));
#19293=DIRECTION('',(0.,0.,-1.));
#19294=DIRECTION('center_axis',(0.866025403784439,-0.5,0.));
#19295=DIRECTION('ref_axis',(-0.5,-0.866025403784439,0.));
#19296=DIRECTION('center_axis',(-2.40370335797945E-16,-1.,0.));
#19297=DIRECTION('ref_axis',(-1.,2.40370335797945E-16,0.));
#19298=DIRECTION('center_axis',(-2.40370335797945E-16,-1.,0.));
#19299=DIRECTION('ref_axis',(-1.,2.40370335797945E-16,0.));
#19300=DIRECTION('',(-1.,2.40370335797945E-16,0.));
#19301=DIRECTION('center_axis',(-0.866025403784439,0.5,0.));
#19302=DIRECTION('ref_axis',(0.5,0.866025403784439,0.));
#19303=DIRECTION('center_axis',(-0.866025403784439,-0.5,0.));
#19304=DIRECTION('ref_axis',(-0.5,0.866025403784439,0.));
#19305=DIRECTION('center_axis',(-2.40370335797945E-16,-1.,0.));
#19306=DIRECTION('ref_axis',(-1.,2.40370335797945E-16,0.));
#19307=DIRECTION('center_axis',(0.,0.,-1.));
#19308=DIRECTION('ref_axis',(-1.,0.,0.));
#19309=DIRECTION('center_axis',(0.,0.,1.));
#19310=DIRECTION('ref_axis',(1.,0.,0.));
#19311=DIRECTION('center_axis',(0.,0.,1.));
#19312=DIRECTION('ref_axis',(1.,0.,0.));
#19313=DIRECTION('',(0.832050294337844,1.01896772969045E-16,-0.554700196225229));
#19314=DIRECTION('center_axis',(0.,0.,1.));
#19315=DIRECTION('ref_axis',(1.,0.,0.));
#19316=DIRECTION('center_axis',(0.,0.,-1.));
#19317=DIRECTION('ref_axis',(1.,0.,0.));
#19318=DIRECTION('center_axis',(0.,0.,-1.));
#19319=DIRECTION('ref_axis',(1.,0.,0.));
#19320=DIRECTION('center_axis',(0.,0.,1.));
#19321=DIRECTION('ref_axis',(1.,0.,0.));
#19322=DIRECTION('',(-0.707106781186548,-8.65956056235494E-17,-0.707106781186547));
#19323=DIRECTION('center_axis',(0.,0.,1.));
#19324=DIRECTION('ref_axis',(1.,0.,0.));
#24581=CARTESIAN_POINT('',(0.,0.,0.));
#24582=CARTESIAN_POINT('Origin',(0.,0.,-0.24));
#24583=CARTESIAN_POINT('',(-0.195553227933509,0.000153074281780883,-0.430479697454243));
#24584=CARTESIAN_POINT('',(-0.195558160953945,0.000205798840386435,-0.44065363587909));
#24585=CARTESIAN_POINT('',(-0.1954,-2.39295984553393E-17,-0.24));
#24586=CARTESIAN_POINT('',(0.0862535085070011,0.17548972741326,-0.453066666666667));
#24587=CARTESIAN_POINT('Ctrl Pts',(-0.195553227933509,0.000153074281780883,
-0.430479697454243));
#24588=CARTESIAN_POINT('Ctrl Pts',(-0.195630430217605,0.00963779447124953,
-0.43102175579123));
#24589=CARTESIAN_POINT('Ctrl Pts',(-0.194998712214993,0.019111688516455,
-0.431563814128216));
#24590=CARTESIAN_POINT('Ctrl Pts',(-0.193622187496123,0.0284754106320751,
-0.432105872465203));
#24591=CARTESIAN_POINT('Ctrl Pts',(-0.184317635852011,0.091769033195883,
-0.435769889334259));
#24592=CARTESIAN_POINT('Ctrl Pts',(-0.140982731022398,0.150028880428339,
-0.439433906203315));
#24593=CARTESIAN_POINT('Ctrl Pts',(-0.0830410591985528,0.177195443378647,
-0.443097923072371));
#24594=CARTESIAN_POINT('Ctrl Pts',(-0.0304934781803096,0.201832930055914,
-0.446420837603803));
#24595=CARTESIAN_POINT('Ctrl Pts',(0.0340678230776199,0.200896926114329,
-0.449743752135234));
#24596=CARTESIAN_POINT('Ctrl Pts',(0.0863544310469484,0.175597323663767,
-0.453066666666667));
#24597=CARTESIAN_POINT('',(-0.0861525859670531,0.175382131162754,-0.453066666666667));
#24598=CARTESIAN_POINT('Origin',(0.,0.,-0.453066666666667));
#24599=CARTESIAN_POINT('Ctrl Pts',(-0.0861525859670524,0.175382131162755,
-0.453066666666667));
#24600=CARTESIAN_POINT('Ctrl Pts',(-0.143832504185423,0.147048149360074,
-0.449402649797611));
#24601=CARTESIAN_POINT('Ctrl Pts',(-0.185985128745257,0.0883085765373875,
-0.445738632928555));
#24602=CARTESIAN_POINT('Ctrl Pts',(-0.194094856498636,0.0249448584907909,
-0.442074616059499));
#24603=CARTESIAN_POINT('Ctrl Pts',(-0.195143228892278,0.0167536127697661,
-0.441600955999363));
#24604=CARTESIAN_POINT('Ctrl Pts',(-0.195622689264249,0.00848509008189603,
-0.441127295939226));
#24605=CARTESIAN_POINT('Ctrl Pts',(-0.195558160953945,0.000205798840386435,
-0.44065363587909));
#24606=CARTESIAN_POINT('Origin',(0.,0.,-0.24));
#24607=CARTESIAN_POINT('',(-0.195096259697753,-1.61683889792347E-5,-0.360479697454244));
#24608=CARTESIAN_POINT('',(-0.1950945860993,3.61475788830789E-6,-0.37065363587909));
#24609=CARTESIAN_POINT('',(-0.1954,-2.39295984553393E-17,-0.24));
#24610=CARTESIAN_POINT('Ctrl Pts',(-0.195096259697753,-1.61683889792347E-5,
-0.360479697454244));
#24611=CARTESIAN_POINT('Ctrl Pts',(-0.195070888875686,0.0332768877299866,
-0.362370987910228));
#24612=CARTESIAN_POINT('Ctrl Pts',(-0.186971229054641,0.0665814795668455,
-0.364262278366212));
#24613=CARTESIAN_POINT('Ctrl Pts',(-0.170868833427777,0.0954169932588536,
-0.366153568822197));
#24614=CARTESIAN_POINT('Ctrl Pts',(-0.139673493218476,0.151280336861681,
-0.369817585691253));
#24615=CARTESIAN_POINT('Ctrl Pts',(-0.078442509106134,0.190370461531553,
-0.373481602560308));
#24616=CARTESIAN_POINT('Ctrl Pts',(-0.0146381891088212,0.195156588972792,
-0.377145619429364));
#24617=CARTESIAN_POINT('Ctrl Pts',(0.0491661308884916,0.199942716414032,
-0.38080963629842));
#24618=CARTESIAN_POINT('Ctrl Pts',(0.115543786770775,0.17042484662664,-0.384473653167476));
#24619=CARTESIAN_POINT('Ctrl Pts',(0.154723399880928,0.119839217267535,
-0.388137670036532));
#24620=CARTESIAN_POINT('Ctrl Pts',(0.193903012991081,0.0692535879084296,
-0.391801686905588));
#24621=CARTESIAN_POINT('Ctrl Pts',(0.205884583329105,-0.00239980102238897,
-0.395465703774644));
#24622=CARTESIAN_POINT('Ctrl Pts',(0.185295223086548,-0.062978599706434,
-0.3991297206437));
#24623=CARTESIAN_POINT('Ctrl Pts',(0.16470586284399,-0.123557398390479,
-0.402793737512756));
#24624=CARTESIAN_POINT('Ctrl Pts',(0.111545572020852,-0.173061606827751,
-0.406457754381811));
#24625=CARTESIAN_POINT('Ctrl Pts',(0.0496553570667544,-0.189298243122558,
-0.410121771250867));
#24626=CARTESIAN_POINT('Ctrl Pts',(-0.012234857887343,-0.205534879417366,
-0.413785788119923));
#24627=CARTESIAN_POINT('Ctrl Pts',(-0.0828549969723998,-0.188503943569709,
-0.417449804988979));
#24628=CARTESIAN_POINT('Ctrl Pts',(-0.130527967285623,-0.145824776698301,
-0.421113821858035));
#24629=CARTESIAN_POINT('Ctrl Pts',(-0.171148150471846,-0.109459608655245,
-0.424235780390105));
#24630=CARTESIAN_POINT('Ctrl Pts',(-0.195108585146772,-0.0544737086663899,
-0.427357738922174));
#24631=CARTESIAN_POINT('Ctrl Pts',(-0.195553227933509,0.000153074281780883,
-0.430479697454243));
#24632=CARTESIAN_POINT('Ctrl Pts',(-0.195558160953945,0.000205798840386435,
-0.44065363587909));
#24633=CARTESIAN_POINT('Ctrl Pts',(-0.1951235278669,-0.0555597077082796,
-0.437463279070171));
#24634=CARTESIAN_POINT('Ctrl Pts',(-0.170009480570289,-0.111813756765947,
-0.434272922261251));
#24635=CARTESIAN_POINT('Ctrl Pts',(-0.12783196242833,-0.14823305616899,
-0.431082565452331));
#24636=CARTESIAN_POINT('Ctrl Pts',(-0.0793925096577201,-0.190059389511667,
-0.427418548583275));
#24637=CARTESIAN_POINT('Ctrl Pts',(-0.00844677316957623,-0.205724192926515,
-0.42375453171422));
#24638=CARTESIAN_POINT('Ctrl Pts',(0.0531396320705838,-0.188335328572067,
-0.420090514845164));
#24639=CARTESIAN_POINT('Ctrl Pts',(0.114726037310744,-0.170946464217619,
-0.416426497976108));
#24640=CARTESIAN_POINT('Ctrl Pts',(0.16695311130292,-0.120503932093875,
-0.412762481107052));
#24641=CARTESIAN_POINT('Ctrl Pts',(0.186420314612119,-0.0595639392003285,
-0.409098464237996));
#24642=CARTESIAN_POINT('Ctrl Pts',(0.205887517921318,0.00137605369321816,
-0.40543444736894));
#24643=CARTESIAN_POINT('Ctrl Pts',(0.192594850547539,0.0728135073565672,
-0.401770430499884));
#24644=CARTESIAN_POINT('Ctrl Pts',(0.152491794432586,0.122672995578315,
-0.398106413630828));
#24645=CARTESIAN_POINT('Ctrl Pts',(0.112388738317632,0.172532483800064,
-0.394442396761773));
#24646=CARTESIAN_POINT('Ctrl Pts',(0.0454752934615041,0.200814006580211,
-0.390778379892717));
#24647=CARTESIAN_POINT('Ctrl Pts',(-0.0182308640572237,0.194851488824733,
-0.387114363023661));
#24648=CARTESIAN_POINT('Ctrl Pts',(-0.0819370215759516,0.188888971069255,
-0.383450346154605));
#24649=CARTESIAN_POINT('Ctrl Pts',(-0.142435891757279,0.148682412778151,
-0.379786329285549));
#24650=CARTESIAN_POINT('Ctrl Pts',(-0.172596664765289,0.092255122594269,
-0.376122312416493));
#24651=CARTESIAN_POINT('Ctrl Pts',(-0.187602009772644,0.0641818713942949,
-0.374299420237359));
#24652=CARTESIAN_POINT('Ctrl Pts',(-0.195098125369958,0.0320936947925797,
-0.372476528058224));
#24653=CARTESIAN_POINT('Ctrl Pts',(-0.1950945860993,3.61475788830789E-6,
-0.37065363587909));
#24654=CARTESIAN_POINT('Origin',(0.,0.,-0.24));
#24655=CARTESIAN_POINT('',(-0.195607476207092,-0.000117485405063567,-0.290479697454244));
#24656=CARTESIAN_POINT('',(-0.195578322079833,-0.0001312749683362,-0.30065363587909));
#24657=CARTESIAN_POINT('',(-0.1954,-2.39295984553393E-17,-0.24));
#24658=CARTESIAN_POINT('Ctrl Pts',(-0.195607476207092,-0.000117485405063567,
-0.290479697454244));
#24659=CARTESIAN_POINT('Ctrl Pts',(-0.195201685186576,0.056545827244161,
-0.293720220029226));
#24660=CARTESIAN_POINT('Ctrl Pts',(-0.169152593581526,0.113534805853513,
-0.296960742604209));
#24661=CARTESIAN_POINT('Ctrl Pts',(-0.12580569557274,0.149911508696811,
-0.300201265179191));
#24662=CARTESIAN_POINT('Ctrl Pts',(-0.0767939198944633,0.191042175055213,
-0.303865282048247));
#24663=CARTESIAN_POINT('Ctrl Pts',(-0.0056677086826894,0.205821011997338,
-0.307529298917303));
#24664=CARTESIAN_POINT('Ctrl Pts',(0.0556722927194857,0.187619627746999,
-0.311193315786359));
#24665=CARTESIAN_POINT('Ctrl Pts',(0.11701229412166,0.169418243496659,-0.314857332655414));
#24666=CARTESIAN_POINT('Ctrl Pts',(0.168566085714236,0.118236638053856,
-0.31852134952447));
#24667=CARTESIAN_POINT('Ctrl Pts',(0.187211386887736,0.0570300966780328,
-0.322185366393526));
#24668=CARTESIAN_POINT('Ctrl Pts',(0.205856688061235,-0.00417644469779128,
-0.325849383262582));
#24669=CARTESIAN_POINT('Ctrl Pts',(0.191593498815658,-0.0754079220066363,
-0.329513400131638));
#24670=CARTESIAN_POINT('Ctrl Pts',(0.150818988166717,-0.124716363406268,
-0.333177417000694));
#24671=CARTESIAN_POINT('Ctrl Pts',(0.110044477517776,-0.174024804805899,
-0.33684143386975));
#24672=CARTESIAN_POINT('Ctrl Pts',(0.0427586454654721,-0.201410210296317,
-0.340505450738806));
#24673=CARTESIAN_POINT('Ctrl Pts',(-0.0208603338378075,-0.19459022297966,
-0.344169467607862));
#24674=CARTESIAN_POINT('Ctrl Pts',(-0.084479313141087,-0.187770235663004,
-0.347833484476918));
#24675=CARTESIAN_POINT('Ctrl Pts',(-0.144431439695342,-0.146744855539273,
-0.351497501345974));
#24676=CARTESIAN_POINT('Ctrl Pts',(-0.17382765481934,-0.0899138842095152,
-0.35516151821503));
#24677=CARTESIAN_POINT('Ctrl Pts',(-0.188050145833162,-0.0624178961840224,
-0.356934244628101));
#24678=CARTESIAN_POINT('Ctrl Pts',(-0.195120040035807,-0.0312220996446506,
-0.358706971041172));
#24679=CARTESIAN_POINT('Ctrl Pts',(-0.195096259697753,-1.61683889792347E-5,
-0.360479697454244));
#24680=CARTESIAN_POINT('Ctrl Pts',(-0.1950945860993,3.61475788830789E-6,
-0.37065363587909));
#24681=CARTESIAN_POINT('Ctrl Pts',(-0.195091011428967,-0.032407429257605,
-0.368812511189169));
#24682=CARTESIAN_POINT('Ctrl Pts',(-0.187437009001129,-0.0648204149726476,
-0.366971386499247));
#24683=CARTESIAN_POINT('Ctrl Pts',(-0.172142443533742,-0.0931006976602427,
-0.365130261809326));
#24684=CARTESIAN_POINT('Ctrl Pts',(-0.141704773459492,-0.149381205654212,
-0.36146624494027));
#24685=CARTESIAN_POINT('Ctrl Pts',(-0.0810067574762996,-0.18929419956549,
-0.357802228071214));
#24686=CARTESIAN_POINT('Ctrl Pts',(-0.0172728534882932,-0.194941042891399,
-0.354138211202158));
#24687=CARTESIAN_POINT('Ctrl Pts',(0.0464610504997132,-0.200587886217307,
-0.350474194333102));
#24688=CARTESIAN_POINT('Ctrl Pts',(0.113230842492533,-0.171968578957846,
-0.346810177464046));
#24689=CARTESIAN_POINT('Ctrl Pts',(0.153090248029826,-0.121917712582769,
-0.34314616059499));
#24690=CARTESIAN_POINT('Ctrl Pts',(0.192949653567118,-0.0718668462076918,
-0.339482143725934));
#24691=CARTESIAN_POINT('Ctrl Pts',(0.205898672648883,-0.000384420716998499,
-0.335818126856879));
#24692=CARTESIAN_POINT('Ctrl Pts',(0.186129314895087,0.0604684215793534,
-0.332154109987823));
#24693=CARTESIAN_POINT('Ctrl Pts',(0.16635995714129,0.121321263875706,-0.328490093118767));
#24694=CARTESIAN_POINT('Ctrl Pts',(0.11387222255193,0.171544522977716,-0.324826076249711));
#24695=CARTESIAN_POINT('Ctrl Pts',(0.0522073964039231,0.188613063308293,
-0.321162059380655));
#24696=CARTESIAN_POINT('Ctrl Pts',(-0.00945742974408397,0.205681603638869,
-0.317498042511599));
#24697=CARTESIAN_POINT('Ctrl Pts',(-0.0802993474507388,0.189595425198011,
-0.313834025642543));
#24698=CARTESIAN_POINT('Ctrl Pts',(-0.128545284234688,0.147569102657344,
-0.310170008773487));
#24699=CARTESIAN_POINT('Ctrl Pts',(-0.170314226307808,0.111184794490457,
-0.306997884475355));
#24700=CARTESIAN_POINT('Ctrl Pts',(-0.195146941473447,0.0553577293133787,
-0.303825760177223));
#24701=CARTESIAN_POINT('Ctrl Pts',(-0.195578322079833,-0.0001312749683362,
-0.30065363587909));
#24702=CARTESIAN_POINT('Origin',(0.,0.,-0.24));
#24703=CARTESIAN_POINT('',(-0.195363183094688,0.000168221922992429,-0.220479697454244));
#24704=CARTESIAN_POINT('',(-0.195397854366554,0.000168478207232705,-0.23065363587909));
#24705=CARTESIAN_POINT('',(-0.1954,-2.39295984553393E-17,-0.24));
#24706=CARTESIAN_POINT('Ctrl Pts',(-0.195363183094688,0.000168221922992429,
-0.220479697454244));
#24707=CARTESIAN_POINT('Ctrl Pts',(-0.195504269673892,0.0164080117818342,
-0.221405435279168));
#24708=CARTESIAN_POINT('Ctrl Pts',(-0.193644174979293,0.032615947390629,
-0.222331173104093));
#24709=CARTESIAN_POINT('Ctrl Pts',(-0.189655926211743,0.0482821032462058,
-0.223256910929018));
#24710=CARTESIAN_POINT('Ctrl Pts',(-0.173870667827724,0.110287843729762,
-0.226920927798073));
#24711=CARTESIAN_POINT('Ctrl Pts',(-0.124747222505265,0.163806438041988,
-0.230584944667129));
#24712=CARTESIAN_POINT('Ctrl Pts',(-0.0643178281358174,0.184834384063959,
-0.234248961536185));
#24713=CARTESIAN_POINT('Ctrl Pts',(-0.00388843376636972,0.205862330085929,
-0.237912978405241));
#24714=CARTESIAN_POINT('Ctrl Pts',(0.0678469096500664,0.194399627817645,
-0.241576995274297));
#24715=CARTESIAN_POINT('Ctrl Pts',(0.11871434919192,0.155587388833047,-0.245241012143353));
#24716=CARTESIAN_POINT('Ctrl Pts',(0.169581788733774,0.116775149848448,
-0.248905029012409));
#24717=CARTESIAN_POINT('Ctrl Pts',(0.199581324401046,0.0506133741475359,
-0.252569045881464));
#24718=CARTESIAN_POINT('Ctrl Pts',(0.195257935435045,-0.0132238767988385,
-0.25623306275052));
#24719=CARTESIAN_POINT('Ctrl Pts',(0.190934546469043,-0.0770611277452132,
-0.259897079619576));
#24720=CARTESIAN_POINT('Ctrl Pts',(0.152288232869768,-0.13857385393705,
-0.263561096488632));
#24721=CARTESIAN_POINT('Ctrl Pts',(0.0966521622178442,-0.170173123868098,
-0.267225113357688));
#24722=CARTESIAN_POINT('Ctrl Pts',(0.04101609156592,-0.201772393799146,
-0.270889130226744));
#24723=CARTESIAN_POINT('Ctrl Pts',(-0.0316097361386534,-0.203458207469406,
-0.2745531470958));
#24724=CARTESIAN_POINT('Ctrl Pts',(-0.088652081273832,-0.174474468983084,
-0.278217163964856));
#24725=CARTESIAN_POINT('Ctrl Pts',(-0.14569442640901,-0.145490730496762,
-0.281881180833912));
#24726=CARTESIAN_POINT('Ctrl Pts',(-0.187153288974794,-0.0858374398538568,
-0.285545197702967));
#24727=CARTESIAN_POINT('Ctrl Pts',(-0.194434050185296,-0.0222695466450644,
-0.289209214572023));
#24728=CARTESIAN_POINT('Ctrl Pts',(-0.195275574921494,-0.014922244211076,
-0.289632708866097));
#24729=CARTESIAN_POINT('Ctrl Pts',(-0.195660507833257,-0.00752264584909209,
-0.29005620316017));
#24730=CARTESIAN_POINT('Ctrl Pts',(-0.195607476207092,-0.000117485405063567,
-0.290479697454244));
#24731=CARTESIAN_POINT('Ctrl Pts',(-0.195578322079833,-0.0001312749683362,
-0.30065363587909));
#24732=CARTESIAN_POINT('Ctrl Pts',(-0.195645215081361,-0.00873580190638232,
-0.300161743308167));
#24733=CARTESIAN_POINT('Ctrl Pts',(-0.195125357252179,-0.0173321998828463,
-0.299669850737243));
#24734=CARTESIAN_POINT('Ctrl Pts',(-0.193990913268632,-0.0258467116936429,
-0.29917795816632));
#24735=CARTESIAN_POINT('Ctrl Pts',(-0.185540649657384,-0.0892697368634882,
-0.295513941297264));
#24736=CARTESIAN_POINT('Ctrl Pts',(-0.142990166573644,-0.148149320562704,
-0.291849924428208));
#24737=CARTESIAN_POINT('Ctrl Pts',(-0.0854237009492422,-0.1760775732527,
-0.288185907559152));
#24738=CARTESIAN_POINT('Ctrl Pts',(-0.0278572353248403,-0.204005825942696,
-0.284521890690096));
#24739=CARTESIAN_POINT('Ctrl Pts',(0.0447252128402237,-0.200982747623472,
-0.28085787382104));
#24740=CARTESIAN_POINT('Ctrl Pts',(0.0997698695794294,-0.168364183330645,
-0.277193856951985));
#24741=CARTESIAN_POINT('Ctrl Pts',(0.154814526318635,-0.135745619037819,
-0.273529840082929));
#24742=CARTESIAN_POINT('Ctrl Pts',(0.192321391631982,-0.0735315687713911,
-0.269865823213873));
#24743=CARTESIAN_POINT('Ctrl Pts',(0.195468343855467,-0.0096255258008377,
-0.266201806344817));
#24744=CARTESIAN_POINT('Ctrl Pts',(0.198615296078951,0.0542805171697163,
-0.262537789475761));
#24745=CARTESIAN_POINT('Ctrl Pts',(0.167402335212573,0.119878552844396,
-0.258873772606705));
#24746=CARTESIAN_POINT('Ctrl Pts',(0.11582871597203,0.157747367680544,-0.255209755737649));
#24747=CARTESIAN_POINT('Ctrl Pts',(0.0642550967314876,0.195616182516693,
-0.251545738868593));
#24748=CARTESIAN_POINT('Ctrl Pts',(-0.00767918088321898,0.20575577651431,
-0.247881721999537));
#24749=CARTESIAN_POINT('Ctrl Pts',(-0.0677110434843187,0.183618459739802,
-0.244217705130482));
#24750=CARTESIAN_POINT('Ctrl Pts',(-0.127742906085418,0.161481142965294,
-0.240553688261426));
#24751=CARTESIAN_POINT('Ctrl Pts',(-0.17587235367291,0.107066915418663,
-0.23688967139237));
#24752=CARTESIAN_POINT('Ctrl Pts',(-0.190512960004344,0.0447809775925131,
-0.233225654523314));
#24753=CARTESIAN_POINT('Ctrl Pts',(-0.193938700459235,0.0302067549031298,
-0.232368314975239));
#24754=CARTESIAN_POINT('Ctrl Pts',(-0.195530898725577,0.0152015494639044,
-0.231510975427165));
#24755=CARTESIAN_POINT('Ctrl Pts',(-0.195397854366554,0.000168478207232705,
-0.23065363587909));
#24756=CARTESIAN_POINT('Origin',(0.,0.,-0.24));
#24757=CARTESIAN_POINT('',(-0.195166600644982,-0.000111941290030684,-0.150479697454244));
#24758=CARTESIAN_POINT('',(-0.195146587185711,-9.71091332246861E-5,-0.16065363587909));
#24759=CARTESIAN_POINT('',(-0.1954,-2.39295984553393E-17,-0.24));
#24760=CARTESIAN_POINT('Ctrl Pts',(-0.195166600644982,-0.000111941290030684,
-0.150479697454244));
#24761=CARTESIAN_POINT('Ctrl Pts',(-0.194952618558542,0.0398988589954238,
-0.152754667398166));
#24762=CARTESIAN_POINT('Ctrl Pts',(-0.182960043012118,0.0800273756788333,
-0.155029637342089));
#24763=CARTESIAN_POINT('Ctrl Pts',(-0.160117027062204,0.112530200621256,
-0.157304607286012));
#24764=CARTESIAN_POINT('Ctrl Pts',(-0.123326564839096,0.164878540079165,
-0.160968624155068));
#24765=CARTESIAN_POINT('Ctrl Pts',(-0.0583904729961102,0.197446125267583,
-0.164632641024124));
#24766=CARTESIAN_POINT('Ctrl Pts',(0.0055670940850077,0.195626035987967,
-0.168296657893179));
#24767=CARTESIAN_POINT('Ctrl Pts',(0.0695246611661256,0.19380594670835,
-0.171960674762235));
#24768=CARTESIAN_POINT('Ctrl Pts',(0.132503703485376,0.157598182960699,
-0.175624691631291));
#24769=CARTESIAN_POINT('Ctrl Pts',(0.166257543654539,0.103242261140942,
-0.179288708500347));
#24770=CARTESIAN_POINT('Ctrl Pts',(0.200011383823701,0.0488863393211846,
-0.182952725369403));
#24771=CARTESIAN_POINT('Ctrl Pts',(0.204540021842776,-0.0236177405706785,
-0.186616742238459));
#24772=CARTESIAN_POINT('Ctrl Pts',(0.17781237832736,-0.0817513731146722,
-0.190280759107515));
#24773=CARTESIAN_POINT('Ctrl Pts',(0.151084734811943,-0.139885005658666,
-0.193944775976571));
#24774=CARTESIAN_POINT('Ctrl Pts',(0.0931008097620331,-0.183648190854791,
-0.197608792845626));
#24775=CARTESIAN_POINT('Ctrl Pts',(0.0298668118705716,-0.193412789202221,
-0.201272809714682));
#24776=CARTESIAN_POINT('Ctrl Pts',(-0.0333671860208894,-0.203177387549652,
-0.204936826583738));
#24777=CARTESIAN_POINT('Ctrl Pts',(-0.101851256753902,-0.178943399048388,
-0.208600843452794));
#24778=CARTESIAN_POINT('Ctrl Pts',(-0.14486975639762,-0.131579961470313,
-0.21226486032185));
#24779=CARTESIAN_POINT('Ctrl Pts',(-0.177019350761991,-0.0961832061569353,
-0.215003139365981));
#24780=CARTESIAN_POINT('Ctrl Pts',(-0.194945857138201,-0.0478681389712799,
-0.217741418410112));
#24781=CARTESIAN_POINT('Ctrl Pts',(-0.195363183094688,0.000168221922992429,
-0.220479697454244));
#24782=CARTESIAN_POINT('Ctrl Pts',(-0.195397854366554,0.000168478207232705,
-0.23065363587909));
#24783=CARTESIAN_POINT('Ctrl Pts',(-0.194962306296955,-0.049045372075947,
-0.227846958558109));
#24784=CARTESIAN_POINT('Ctrl Pts',(-0.176037076517356,-0.0985578644675523,
-0.225040281237128));
#24785=CARTESIAN_POINT('Ctrl Pts',(-0.142421832474098,-0.134225725993483,
-0.222233603916146));
#24786=CARTESIAN_POINT('Ctrl Pts',(-0.0985383335370456,-0.180788843647661,
-0.21856958704709));
#24787=CARTESIAN_POINT('Ctrl Pts',(-0.0296195705875667,-0.203757430850347,
-0.214905570178034));
#24788=CARTESIAN_POINT('Ctrl Pts',(0.0334238616745515,-0.19282989819453,
-0.211241553308979));
#24789=CARTESIAN_POINT('Ctrl Pts',(0.0964672939366692,-0.181902365538714,
-0.207577536439923));
#24790=CARTESIAN_POINT('Ctrl Pts',(0.153635395511427,-0.137078713024395,
-0.203913519570867));
#24791=CARTESIAN_POINT('Ctrl Pts',(0.179287838103686,-0.0784626953524838,
-0.200249502701811));
#24792=CARTESIAN_POINT('Ctrl Pts',(0.204940280695945,-0.0198466776805732,
-0.196585485832755));
#24793=CARTESIAN_POINT('Ctrl Pts',(0.199077064305706,0.0525617051489285,
-0.192921468963699));
#24794=CARTESIAN_POINT('Ctrl Pts',(0.164327880102392,0.106286744317414,
-0.189257452094643));
#24795=CARTESIAN_POINT('Ctrl Pts',(0.129578695899078,0.160011783485899,
-0.185593435225588));
#24796=CARTESIAN_POINT('Ctrl Pts',(0.0659435438826869,0.195053478993368,
-0.181929418356532));
#24797=CARTESIAN_POINT('Ctrl Pts',(0.00196328933688991,0.195695351501948,
-0.178265401487476));
#24798=CARTESIAN_POINT('Ctrl Pts',(-0.0620169652089071,0.196337224010529,
-0.17460138461842));
#24799=CARTESIAN_POINT('Ctrl Pts',(-0.12634232228411,0.162579273520222,
-0.170937367749364));
#24800=CARTESIAN_POINT('Ctrl Pts',(-0.162162389583139,0.109562219268833,
-0.167273350880308));
#24801=CARTESIAN_POINT('Ctrl Pts',(-0.183734218654723,0.0776338919811593,
-0.165066779213235));
#24802=CARTESIAN_POINT('Ctrl Pts',(-0.194967807817681,0.0387207125249729,
-0.162860207546163));
#24803=CARTESIAN_POINT('Ctrl Pts',(-0.195146587185711,-9.71091332246862E-5,
-0.16065363587909));
#24804=CARTESIAN_POINT('Origin',(0.,0.,-0.24));
#24805=CARTESIAN_POINT('',(-0.195709073584005,-9.38010969637637E-6,-0.0804796974542435));
#24806=CARTESIAN_POINT('',(-0.195698342875023,-3.28562868159645E-5,-0.0906536358790898));
#24807=CARTESIAN_POINT('',(-0.1954,-2.39295984553393E-17,-0.24));
#24808=CARTESIAN_POINT('Ctrl Pts',(-0.195709144608334,-9.38226522190222E-6,
-0.0804796974542435));
#24809=CARTESIAN_POINT('Ctrl Pts',(-0.195653902033672,0.0632821337469015,
-0.0841038995171643));
#24810=CARTESIAN_POINT('Ctrl Pts',(-0.162090188595658,0.126619703158733,
-0.0877281015800852));
#24811=CARTESIAN_POINT('Ctrl Pts',(-0.109671443000727,0.162085329147497,
-0.0913523036430061));
#24812=CARTESIAN_POINT('Ctrl Pts',(-0.0566768348690305,0.197940573871278,
-0.0950163205120619));
#24813=CARTESIAN_POINT('Ctrl Pts',(0.015589356712093,0.205308119443704,
-0.0986803373811178));
#24814=CARTESIAN_POINT('Ctrl Pts',(0.0747239197390152,0.18087830035279,
-0.102344354250174));
#24815=CARTESIAN_POINT('Ctrl Pts',(0.133858482765937,0.156448481261876,
-0.106008371119229));
#24816=CARTESIAN_POINT('Ctrl Pts',(0.179861417238658,0.100221297507622,
-0.109672387988285));
#24817=CARTESIAN_POINT('Ctrl Pts',(0.1920954828139,0.0374178292863625,-0.113336404857341));
#24818=CARTESIAN_POINT('Ctrl Pts',(0.204329548389143,-0.0253856389348972,
-0.117000421726397));
#24819=CARTESIAN_POINT('Ctrl Pts',(0.182794745066906,-0.0947653916231622,
-0.120664438595453));
#24820=CARTESIAN_POINT('Ctrl Pts',(0.137151991839732,-0.139605522577995,
-0.124328455464509));
#24821=CARTESIAN_POINT('Ctrl Pts',(0.0915092386125581,-0.184445653532828,
-0.127992472333565));
#24822=CARTESIAN_POINT('Ctrl Pts',(0.0217585354804476,-0.20474616275423,
-0.13165648920262));
#24823=CARTESIAN_POINT('Ctrl Pts',(-0.0408176472256261,-0.191401359750901,
-0.135320506071676));
#24824=CARTESIAN_POINT('Ctrl Pts',(-0.1033938299317,-0.178056556747573,
-0.138984522940732));
#24825=CARTESIAN_POINT('Ctrl Pts',(-0.158795492211738,-0.131066441519513,
-0.142648539809788));
#24826=CARTESIAN_POINT('Ctrl Pts',(-0.182173907050141,-0.0715068370417835,
-0.146312556678844));
#24827=CARTESIAN_POINT('Ctrl Pts',(-0.191036779795085,-0.0489274962749229,
-0.147701603603977));
#24828=CARTESIAN_POINT('Ctrl Pts',(-0.195297253430087,-0.0245416614527496,
-0.14909065052911));
#24829=CARTESIAN_POINT('Ctrl Pts',(-0.195166600644982,-0.000111941290030684,
-0.150479697454244));
#24830=CARTESIAN_POINT('Ctrl Pts',(-0.195146587185711,-9.71091332246862E-5,
-0.16065363587909));
#24831=CARTESIAN_POINT('Ctrl Pts',(-0.19526467133228,-0.0257363615406621,
-0.159196190677107));
#24832=CARTESIAN_POINT('Ctrl Pts',(-0.190559950845405,-0.0513340128677999,
-0.157738745475124));
#24833=CARTESIAN_POINT('Ctrl Pts',(-0.18082594422566,-0.0748498819709867,
-0.15628130027314));
#24834=CARTESIAN_POINT('Ctrl Pts',(-0.156354654046297,-0.133968770946947,
-0.152617283404085));
#24835=CARTESIAN_POINT('Ctrl Pts',(-0.100097296164716,-0.179930390886395,
-0.148953266535029));
#24836=CARTESIAN_POINT('Ctrl Pts',(-0.037285810874828,-0.192120531087848,
-0.145289249665973));
#24837=CARTESIAN_POINT('Ctrl Pts',(0.0255256744150603,-0.204310671289302,
-0.141625232796917));
#24838=CARTESIAN_POINT('Ctrl Pts',(0.0948912871132562,-0.182729331752761,
-0.137961215927861));
#24839=CARTESIAN_POINT('Ctrl Pts',(0.139700179401184,-0.137056046072734,
-0.134297199058805));
#24840=CARTESIAN_POINT('Ctrl Pts',(0.184509071689111,-0.0913827603927075,
-0.130633182189749));
#24841=CARTESIAN_POINT('Ctrl Pts',(0.20476124356677,-0.0216175285691954,
-0.126969165320693));
#24842=CARTESIAN_POINT('Ctrl Pts',(0.191373133778922,0.040949670807561,
-0.123305148451638));
#24843=CARTESIAN_POINT('Ctrl Pts',(0.177985023991073,0.103516870184318,
-0.119641131582582));
#24844=CARTESIAN_POINT('Ctrl Pts',(0.130956632537716,0.158886037114319,
-0.115977114713526));
#24845=CARTESIAN_POINT('Ctrl Pts',(0.0713811391615662,0.182223175406547,
-0.11231309784447));
#24846=CARTESIAN_POINT('Ctrl Pts',(0.011805645785417,0.205560313698776,
-0.108649080975414));
#24847=CARTESIAN_POINT('Ctrl Pts',(-0.0603169495135242,0.196865423353232,
-0.104985064106358));
#24848=CARTESIAN_POINT('Ctrl Pts',(-0.112640228305471,0.160039184697078,
-0.101321047237302));
#24849=CARTESIAN_POINT('Ctrl Pts',(-0.163418191256275,0.124300572261585,
-0.0977652434512315));
#24850=CARTESIAN_POINT('Ctrl Pts',(-0.195549073724041,0.062067736358378,
-0.0942094396651606));
#24851=CARTESIAN_POINT('Ctrl Pts',(-0.195698342875023,-3.28562868159645E-5,
-0.0906536358790898));
#24852=CARTESIAN_POINT('Origin',(0.,0.,-0.582472289227037));
#24853=CARTESIAN_POINT('',(-0.155796097460729,-7.46884010135441E-6,-0.0574722892270367));
#24854=CARTESIAN_POINT('',(-0.155389280676728,9.5162621374309E-5,-0.0436610441062962));
#24855=CARTESIAN_POINT('',(-0.15555,-2.84370958922189E-15,-0.582472289227037));
#24856=CARTESIAN_POINT('',(0.150444513166827,-0.0404002418790732,-0.0254000000000001));
#24857=CARTESIAN_POINT('Ctrl Pts',(-0.155796097460729,-7.46884010136202E-6,
-0.0574722892270367));
#24858=CARTESIAN_POINT('Ctrl Pts',(-0.155796580576894,-0.000560975889831939,
-0.0574324744209017));
#24859=CARTESIAN_POINT('Ctrl Pts',(-0.155542040915253,-0.0520513824587016,
-0.0537286427457109));
#24860=CARTESIAN_POINT('Ctrl Pts',(-0.0993493656725074,-0.153895266515289,
-0.0463607942014641));
#24861=CARTESIAN_POINT('Ctrl Pts',(0.068138238496685,-0.167299521168177,
-0.0357098459319202));
#24862=CARTESIAN_POINT('Ctrl Pts',(0.138167064954546,-0.0849802566602034,
-0.0287229145314322));
#24863=CARTESIAN_POINT('Ctrl Pts',(0.150444513166827,-0.0404002418790733,
-0.0254000000000001));
#24864=CARTESIAN_POINT('',(0.0106175386826097,-0.155187210724091,-0.0254000000000001));
#24865=CARTESIAN_POINT('Origin',(0.,0.,-0.0254000000000001));
#24866=CARTESIAN_POINT('Ctrl Pts',(-0.155389280676728,9.51626213743055E-5,
-0.0436610441062962));
#24867=CARTESIAN_POINT('Ctrl Pts',(-0.15512974883406,-0.0338312999427815,
-0.0412380462732533));
#24868=CARTESIAN_POINT('Ctrl Pts',(-0.127591546791687,-0.119392150871042,
-0.0351510315711546));
#24869=CARTESIAN_POINT('Ctrl Pts',(-0.0404206461299352,-0.158679121552366,
-0.029064016869056));
#24870=CARTESIAN_POINT('Ctrl Pts',(0.0106175386826097,-0.155187210724091,
-0.0254000000000001));
#24871=CARTESIAN_POINT('Origin',(0.,0.,-0.582472289227037));
#24872=CARTESIAN_POINT('',(-0.155364200257559,-8.91119123082438E-5,-0.127472289227037));
#24873=CARTESIAN_POINT('',(-0.155787498639764,-2.6155554834012E-5,-0.113661044106296));
#24874=CARTESIAN_POINT('',(-0.15555,-2.84370958922189E-15,-0.582472289227037));
#24875=CARTESIAN_POINT('Ctrl Pts',(-0.155364200257559,-8.91119123082353E-5,
-0.127472289227037));
#24876=CARTESIAN_POINT('Ctrl Pts',(-0.155468207630757,-0.0195366194420458,
-0.126083242301904));
#24877=CARTESIAN_POINT('Ctrl Pts',(-0.143130308880635,-0.0901555192989463,
-0.121030178507715));
#24878=CARTESIAN_POINT('Ctrl Pts',(-0.038204614525159,-0.179150510879271,
-0.11231309784447));
#24879=CARTESIAN_POINT('Ctrl Pts',(0.128372486890396,-0.130669279414751,
-0.101321047237302));
#24880=CARTESIAN_POINT('Ctrl Pts',(0.179801432490814,0.0350219262760309,
-0.0903289966301345));
#24881=CARTESIAN_POINT('Ctrl Pts',(0.0699382320215437,0.169302454929678,
-0.0793369460229671));
#24882=CARTESIAN_POINT('Ctrl Pts',(-0.10202117751736,0.151771175659713,
-0.0683847102219343));
#24883=CARTESIAN_POINT('Ctrl Pts',(-0.1557521210918,0.050376335231986,-0.0610964912899576));
#24884=CARTESIAN_POINT('Ctrl Pts',(-0.155796097460729,-7.46884010136202E-6,
-0.0574722892270367));
#24885=CARTESIAN_POINT('Ctrl Pts',(-0.155787498639764,-2.61555548340198E-5,
-0.113661044106296));
#24886=CARTESIAN_POINT('Ctrl Pts',(-0.155791114881889,-0.00153062434586674,
-0.113552831023311));
#24887=CARTESIAN_POINT('Ctrl Pts',(-0.155095219214847,-0.0539719215336349,
-0.10978060107127));
#24888=CARTESIAN_POINT('Ctrl Pts',(-0.0965231054289514,-0.155685461973447,
-0.102344354250173));
#24889=CARTESIAN_POINT('Ctrl Pts',(0.0766264864264418,-0.166372403162464,
-0.091352303643006));
#24890=CARTESIAN_POINT('Ctrl Pts',(0.181065301238179,-0.0278415620581252,
-0.0803602530358381));
#24891=CARTESIAN_POINT('Ctrl Pts',(0.123039270360697,0.135703326763709,
-0.0693682024286707));
#24892=CARTESIAN_POINT('Ctrl Pts',(-0.0452659821533855,0.177444214884968,
-0.058376151821503));
#24893=CARTESIAN_POINT('Ctrl Pts',(-0.144950921528674,0.0860145677096474,
-0.0498070990473782));
#24894=CARTESIAN_POINT('Ctrl Pts',(-0.155522208553431,0.017471730314721,
-0.0449020631423093));
#24895=CARTESIAN_POINT('Ctrl Pts',(-0.155389280676728,9.51626213743055E-5,
-0.0436610441062962));
#24896=CARTESIAN_POINT('Origin',(0.,0.,-0.582472289227037));
#24897=CARTESIAN_POINT('',(-0.155520691557721,0.000133914637262764,-0.197472289227037));
#24898=CARTESIAN_POINT('',(-0.155348268355872,-7.73046349714923E-5,-0.183661044106296));
#24899=CARTESIAN_POINT('',(-0.15555,-2.84370958922189E-15,-0.582472289227037));
#24900=CARTESIAN_POINT('Ctrl Pts',(-0.155520691557721,0.000133914637262762,
-0.197472289227037));
#24901=CARTESIAN_POINT('Ctrl Pts',(-0.155188475321633,-0.0381058803325632,
-0.194734010182906));
#24902=CARTESIAN_POINT('Ctrl Pts',(-0.121822858612577,-0.128032047716084,
-0.188331714269719));
#24903=CARTESIAN_POINT('Ctrl Pts',(0.0279551249589101,-0.181032955704809,
-0.178265401487475));
#24904=CARTESIAN_POINT('Ctrl Pts',(0.166431064695553,-0.0765186753989169,
-0.167273350880308));
#24905=CARTESIAN_POINT('Ctrl Pts',(0.15561587057272,0.0966339800849018,
-0.15628130027314));
#24906=CARTESIAN_POINT('Ctrl Pts',(0.00521070118542118,0.183104568379892,
-0.145289249665973));
#24907=CARTESIAN_POINT('Ctrl Pts',(-0.130271184964665,0.115155947767654,
-0.135686245983938));
#24908=CARTESIAN_POINT('Ctrl Pts',(-0.15519385781362,0.03176186037225,-0.12974725917096));
#24909=CARTESIAN_POINT('Ctrl Pts',(-0.155364200257559,-8.91119123082353E-5,
-0.127472289227037));
#24910=CARTESIAN_POINT('Ctrl Pts',(-0.155348268355872,-7.73046349714958E-5,
-0.183661044106296));
#24911=CARTESIAN_POINT('Ctrl Pts',(-0.155442270346654,-0.0204876716358764,
-0.182203598904313));
#24912=CARTESIAN_POINT('Ctrl Pts',(-0.142281509160764,-0.0920933232311109,
-0.177082136833274));
#24913=CARTESIAN_POINT('Ctrl Pts',(-0.0348991934490358,-0.179823450787922,
-0.168296657893179));
#24914=CARTESIAN_POINT('Ctrl Pts',(0.130758243427182,-0.128283368419821,
-0.157304607286012));
#24915=CARTESIAN_POINT('Ctrl Pts',(0.179124036706147,0.0383284300983071,
-0.146312556678844));
#24916=CARTESIAN_POINT('Ctrl Pts',(0.0668118623371123,0.17055986176609,
-0.135320506071676));
#24917=CARTESIAN_POINT('Ctrl Pts',(-0.103734078699234,0.149999339088803,
-0.124436668547494));
#24918=CARTESIAN_POINT('Ctrl Pts',(-0.155668671534159,0.0494096028175303,
-0.117216847892367));
#24919=CARTESIAN_POINT('Ctrl Pts',(-0.155787498639764,-2.61555548340198E-5,
-0.113661044106296));
#24920=CARTESIAN_POINT('Origin',(0.,0.,-0.582472289227037));
#24921=CARTESIAN_POINT('',(-0.155715163377754,-9.35253570008701E-5,-0.267472289227037));
#24922=CARTESIAN_POINT('',(-0.155548291948401,0.000134118654731868,-0.253661044106296));
#24923=CARTESIAN_POINT('',(-0.15555,-2.84370958922189E-15,-0.582472289227037));
#24924=CARTESIAN_POINT('Ctrl Pts',(-0.155715163377754,-9.35253570008522E-5,
-0.267472289227037));
#24925=CARTESIAN_POINT('Ctrl Pts',(-0.155757379700425,-0.00598847268079084,
-0.267048794932964));
#24926=CARTESIAN_POINT('Ctrl Pts',(-0.152799763003076,-0.0628429920017419,
-0.262961283769834));
#24927=CARTESIAN_POINT('Ctrl Pts',(-0.0829776968055973,-0.163306819284929,
-0.255209755737649));
#24928=CARTESIAN_POINT('Ctrl Pts',(0.0904657141377962,-0.159280796003317,
-0.244217705130481));
#24929=CARTESIAN_POINT('Ctrl Pts',(0.182759993774958,-0.0123774506736319,
-0.233225654523314));
#24930=CARTESIAN_POINT('Ctrl Pts',(0.111115759797821,0.145628652861839,
-0.222233603916146));
#24931=CARTESIAN_POINT('Ctrl Pts',(-0.0602010160736213,0.173003627342364,
-0.211241553308979));
#24932=CARTESIAN_POINT('Ctrl Pts',(-0.148291552645345,0.0770314971592852,
-0.202987781745942));
#24933=CARTESIAN_POINT('Ctrl Pts',(-0.15563300485043,0.0130617514465919,
-0.198398027051962));
#24934=CARTESIAN_POINT('Ctrl Pts',(-0.155520691557721,0.000133914637262762,
-0.197472289227037));
#24935=CARTESIAN_POINT('Ctrl Pts',(-0.155548291948401,0.00013411865473186,
-0.253661044106296));
#24936=CARTESIAN_POINT('Ctrl Pts',(-0.155201569828512,-0.0390430277707979,
-0.250854366785315));
#24937=CARTESIAN_POINT('Ctrl Pts',(-0.120468353035836,-0.129912631585972,
-0.244383672595278));
#24938=CARTESIAN_POINT('Ctrl Pts',(0.031284490132526,-0.180487370051941,
-0.234248961536185));
#24939=CARTESIAN_POINT('Ctrl Pts',(0.167812098115434,-0.0734405049249859,
-0.223256910929018));
#24940=CARTESIAN_POINT('Ctrl Pts',(0.15380969315891,0.0994836089306307,
-0.21226486032185));
#24941=CARTESIAN_POINT('Ctrl Pts',(0.00183761696418741,0.183169418595726,
-0.201272809714682));
#24942=CARTESIAN_POINT('Ctrl Pts',(-0.131414133088497,0.113238893752059,
-0.191738204309498));
#24943=CARTESIAN_POINT('Ctrl Pts',(-0.155205949365611,0.0308239858406309,
-0.185867615773369));
#24944=CARTESIAN_POINT('Ctrl Pts',(-0.155348268355872,-7.73046349714958E-5,
-0.183661044106296));
#24945=CARTESIAN_POINT('Origin',(0.,0.,-0.582472289227037));
#24946=CARTESIAN_POINT('',(-0.155308204687746,-1.28709974709959E-5,-0.337472289227037));
#24947=CARTESIAN_POINT('',(-0.15569195496171,-0.000104502667989975,-0.323661044106296));
#24948=CARTESIAN_POINT('',(-0.15555,-2.84370958922189E-15,-0.582472289227037));
#24949=CARTESIAN_POINT('Ctrl Pts',(-0.155308204687746,-1.28709974709911E-5,
-0.337472289227037));
#24950=CARTESIAN_POINT('Ctrl Pts',(-0.155327135248565,-0.0248546448297111,
-0.335699562813965));
#24951=CARTESIAN_POINT('Ctrl Pts',(-0.138066551401952,-0.101016698517625,
-0.330262819531838));
#24952=CARTESIAN_POINT('Ctrl Pts',(-0.0195250965894654,-0.182134892710474,
-0.321162059380655));
#24953=CARTESIAN_POINT('Ctrl Pts',(0.141165453703306,-0.116733667162349,
-0.310170008773487));
#24954=CARTESIAN_POINT('Ctrl Pts',(0.175228489841733,0.0533797867075198,
-0.29917795816632));
#24955=CARTESIAN_POINT('Ctrl Pts',(0.052108853983618,0.175610575755033,
-0.288185907559152));
#24956=CARTESIAN_POINT('Ctrl Pts',(-0.111208875107151,0.141675883510508,
-0.277617351246058));
#24957=CARTESIAN_POINT('Ctrl Pts',(-0.155392129635476,0.0450138353522466,
-0.270712811802019));
#24958=CARTESIAN_POINT('Ctrl Pts',(-0.155715163377754,-9.35253570008522E-5,
-0.267472289227037));
#24959=CARTESIAN_POINT('Ctrl Pts',(-0.15569195496171,-0.000104502667989961,
-0.323661044106296));
#24960=CARTESIAN_POINT('Ctrl Pts',(-0.155745205762056,-0.00695421692189423,
-0.323169151535373));
#24961=CARTESIAN_POINT('Ctrl Pts',(-0.152248767557636,-0.0647715135328056,
-0.319013242095394));
#24962=CARTESIAN_POINT('Ctrl Pts',(-0.0799559507003814,-0.164807298147092,
-0.311193315786359));
#24963=CARTESIAN_POINT('Ctrl Pts',(0.0933838621769322,-0.157587648721984,
-0.300201265179191));
#24964=CARTESIAN_POINT('Ctrl Pts',(0.182956936375875,-0.00900941659901149,
-0.289209214572024));
#24965=CARTESIAN_POINT('Ctrl Pts',(0.108414826916839,0.14765037535385,-0.278217163964856));
#24966=CARTESIAN_POINT('Ctrl Pts',(-0.0633770392495001,0.17186553164345,
-0.267225113357688));
#24967=CARTESIAN_POINT('Ctrl Pts',(-0.148969863825595,0.0750959307795305,
-0.259039740071501));
#24968=CARTESIAN_POINT('Ctrl Pts',(-0.155654203156415,0.0121013358193961,
-0.254518383654371));
#24969=CARTESIAN_POINT('Ctrl Pts',(-0.155548291948401,0.00013411865473186,
-0.253661044106296));
#24970=CARTESIAN_POINT('Origin',(0.,0.,-0.582472289227037));
#24971=CARTESIAN_POINT('',(-0.155671978531511,0.000121856215612283,-0.407472289227037));
#24972=CARTESIAN_POINT('',(-0.155306872404023,2.8775618683835E-6,-0.393661044106296));
#24973=CARTESIAN_POINT('',(-0.15555,-2.84370958922189E-15,-0.582472289227037));
#24974=CARTESIAN_POINT('Ctrl Pts',(-0.155671978531511,0.000121856215612291,
-0.407472289227037));
#24975=CARTESIAN_POINT('Ctrl Pts',(-0.15531801647687,-0.0433643059521865,
-0.404350330694967));
#24976=CARTESIAN_POINT('Ctrl Pts',(-0.113858398180907,-0.138508424000405,
-0.397564355293842));
#24977=CARTESIAN_POINT('Ctrl Pts',(0.0464781498992043,-0.177175601660564,
-0.38711436302366));
#24978=CARTESIAN_POINT('Ctrl Pts',(0.17343439203133,-0.0589507354003139,
-0.376122312416494));
#24979=CARTESIAN_POINT('Ctrl Pts',(0.144820268191827,0.112170318563691,
-0.365130261809325));
#24980=CARTESIAN_POINT('Ctrl Pts',(-0.0137013956641988,0.182664248636804,
-0.354138211202158));
#24981=CARTESIAN_POINT('Ctrl Pts',(-0.136348787789886,0.104365623877948,
-0.344918887008062));
#24982=CARTESIAN_POINT('Ctrl Pts',(-0.155288008007231,0.0264903781289625,
-0.339363579683021));
#24983=CARTESIAN_POINT('Ctrl Pts',(-0.155308204687746,-1.28709974709911E-5,
-0.337472289227037));
#24984=CARTESIAN_POINT('Ctrl Pts',(-0.155306872404023,2.87756186839044E-6,
-0.393661044106296));
#24985=CARTESIAN_POINT('Ctrl Pts',(-0.155304026754226,-0.0257982375691955,
-0.391819919416375));
#24986=CARTESIAN_POINT('Ctrl Pts',(-0.137085244699405,-0.102950698396822,
-0.386314777857398));
#24987=CARTESIAN_POINT('Ctrl Pts',(-0.016166963865162,-0.182462532985216,
-0.377145619429364));
#24988=CARTESIAN_POINT('Ctrl Pts',(0.143291190860782,-0.114114530259385,
-0.366153568822197));
#24989=CARTESIAN_POINT('Ctrl Pts',(0.174215754599295,0.0565982325616605,
-0.35516151821503));
#24990=CARTESIAN_POINT('Ctrl Pts',(0.0488656965331514,0.176540319869506,
-0.344169467607861));
#24991=CARTESIAN_POINT('Ctrl Pts',(-0.112746501248559,0.139842800436154,
-0.333669309571618));
#24992=CARTESIAN_POINT('Ctrl Pts',(-0.155348550389943,0.0440680388674291,
-0.326833168404429));
#24993=CARTESIAN_POINT('Ctrl Pts',(-0.15569195496171,-0.000104502667989961,
-0.323661044106296));
#24994=CARTESIAN_POINT('Origin',(2.59090492670967E-17,0.,-0.0254000000000001));
#24995=CARTESIAN_POINT('',(-0.044842238767986,0.190184998415424,-0.0254000000000001));
#24996=CARTESIAN_POINT('Ctrl Pts',(0.150444513166827,-0.0404002418790722,
-0.0254));
#24997=CARTESIAN_POINT('Ctrl Pts',(0.152288523601877,-0.0359477914915009,
-0.0254));
#24998=CARTESIAN_POINT('Ctrl Pts',(0.153909584332356,-0.0314161192062029,
-0.0254));
#24999=CARTESIAN_POINT('Ctrl Pts',(0.155297293824378,-0.0268185318320736,
-0.0254));
#25000=CARTESIAN_POINT('Ctrl Pts',(0.157109245974868,-0.0208153961775976,
-0.0254));
#25001=CARTESIAN_POINT('Ctrl Pts',(0.158523650087112,-0.0146999624105404,
-0.0254));
#25002=CARTESIAN_POINT('Ctrl Pts',(0.159556946383489,-0.00850639978364366,
-0.0254));
#25003=CARTESIAN_POINT('Ctrl Pts',(0.160489936122728,-0.00291407316784563,
-0.0254));
#25004=CARTESIAN_POINT('Ctrl Pts',(0.161111867808762,0.00274714571770028,
-0.0254000000000003));
#25005=CARTESIAN_POINT('Ctrl Pts',(0.161430884359787,0.00842270596691387,
-0.0254000000000002));
#25006=CARTESIAN_POINT('Ctrl Pts',(0.161919051332622,0.0171075878550349,
-0.0254000000000001));
#25007=CARTESIAN_POINT('Ctrl Pts',(0.161701943773179,0.0258371679676822,
-0.0254000000000001));
#25008=CARTESIAN_POINT('Ctrl Pts',(0.160816263117086,0.0345264326241675,
-0.0254000000000001));
#25009=CARTESIAN_POINT('Ctrl Pts',(0.160262807613304,0.0399562919248784,
-0.0254000000000001));
#25010=CARTESIAN_POINT('Ctrl Pts',(0.159446308044253,0.0453760768932331,
-0.0254000000000002));
#25011=CARTESIAN_POINT('Ctrl Pts',(0.158380032328247,0.0507336350772083,
-0.0254000000000001));
#25012=CARTESIAN_POINT('Ctrl Pts',(0.156098217349856,0.0621987339519919,
-0.0254000000000001));
#25013=CARTESIAN_POINT('Ctrl Pts',(0.152675969965111,0.0734017680619525,
-0.0254));
#25014=CARTESIAN_POINT('Ctrl Pts',(0.148188225310357,0.084152422306617,
-0.0254));
#25015=CARTESIAN_POINT('Ctrl Pts',(0.146120109284199,0.0891067149514794,
-0.0254));
#25016=CARTESIAN_POINT('Ctrl Pts',(0.143824981035637,0.093965065234332,
-0.0254000000000001));
#25017=CARTESIAN_POINT('Ctrl Pts',(0.14130650146901,0.0987086415880662,
-0.0254000000000001));
#25018=CARTESIAN_POINT('Ctrl Pts',(0.13912884558959,0.102810273808185,-0.0254000000000001));
#25019=CARTESIAN_POINT('Ctrl Pts',(0.136781562604662,0.106829358853639,
-0.0253999999999999));
#25020=CARTESIAN_POINT('Ctrl Pts',(0.134281947115991,0.110730142526631,
-0.0253999999999999));
#25021=CARTESIAN_POINT('Ctrl Pts',(0.130254692328574,0.117014889037818,
-0.0253999999999999));
#25022=CARTESIAN_POINT('Ctrl Pts',(0.125827047154186,0.123004551843775,
-0.0254));
#25023=CARTESIAN_POINT('Ctrl Pts',(0.121015339265292,0.128651930926206,
-0.0254));
#25024=CARTESIAN_POINT('Ctrl Pts',(0.115989939416535,0.134550114823078,
-0.0254));
#25025=CARTESIAN_POINT('Ctrl Pts',(0.110545683683119,0.140075249109618,
-0.0254000000000001));
#25026=CARTESIAN_POINT('Ctrl Pts',(0.104735241535896,0.145219293087094,
-0.0254000000000001));
#25027=CARTESIAN_POINT('Ctrl Pts',(0.101154909616182,0.148388997626321,
-0.0254000000000001));
#25028=CARTESIAN_POINT('Ctrl Pts',(0.09743534991764,0.151413906784189,-0.0254));
#25029=CARTESIAN_POINT('Ctrl Pts',(0.0935873754776157,0.154290981378466,
-0.0254));
#25030=CARTESIAN_POINT('Ctrl Pts',(0.0905644815369063,0.156551155268278,
-0.0253999999999999));
#25031=CARTESIAN_POINT('Ctrl Pts',(0.0874690119107099,0.158714939473109,
-0.0253999999999999));
#25032=CARTESIAN_POINT('Ctrl Pts',(0.0843113769815779,0.16077906433524,
-0.0253999999999999));
#25033=CARTESIAN_POINT('Ctrl Pts',(0.0749099637749328,0.166924705352815,
-0.0253999999999999));
#25034=CARTESIAN_POINT('Ctrl Pts',(0.0649487520954266,0.172196873794768,
-0.0254000000000001));
#25035=CARTESIAN_POINT('Ctrl Pts',(0.0545782856068879,0.17657123368835,
-0.0254000000000002));
#25036=CARTESIAN_POINT('Ctrl Pts',(0.0469628838054677,0.179783481493254,
-0.0254000000000003));
#25037=CARTESIAN_POINT('Ctrl Pts',(0.0391259623884753,0.182511210134655,
-0.0254));
#25038=CARTESIAN_POINT('Ctrl Pts',(0.0311192198383689,0.18473535989345,
-0.0254));
#25039=CARTESIAN_POINT('Ctrl Pts',(0.0279473244497433,0.185616463578174,
-0.0254));
#25040=CARTESIAN_POINT('Ctrl Pts',(0.0247505316468867,0.186417770388197,
-0.0254));
#25041=CARTESIAN_POINT('Ctrl Pts',(0.0215412556878254,0.187136369631423,
-0.0254));
#25042=CARTESIAN_POINT('Ctrl Pts',(0.00902611956062844,0.189938673784945,
-0.0254));
#25043=CARTESIAN_POINT('Ctrl Pts',(-0.00371436117299067,0.191497453815457,
-0.0254000000000002));
#25044=CARTESIAN_POINT('Ctrl Pts',(-0.0164851355348781,0.191763125459253,
-0.0254000000000003));
#25045=CARTESIAN_POINT('Ctrl Pts',(-0.0259446175737208,0.191959911971292,
-0.0254000000000003));
#25046=CARTESIAN_POINT('Ctrl Pts',(-0.0354216684714881,0.19144650970575,
-0.0254000000000001));
#25047=CARTESIAN_POINT('Ctrl Pts',(-0.044842238767986,0.190184998415424,
-0.0254000000000001));
#25048=CARTESIAN_POINT('',(-0.1954,-2.39295984553393E-17,-0.0254000000000001));
#25049=CARTESIAN_POINT('Origin',(0.,0.,-0.0254000000000001));
#25050=CARTESIAN_POINT('',(-0.178079963314484,0.080770315425888,-0.0254000000000001));
#25051=CARTESIAN_POINT('Origin',(0.,0.,-0.0254000000000001));
#25052=CARTESIAN_POINT('Ctrl Pts',(-0.178226250896966,0.0807893643570701,
-0.0254000000000002));
#25053=CARTESIAN_POINT('Ctrl Pts',(-0.180177392099784,0.0751485900811471,
-0.0254000000000002));
#25054=CARTESIAN_POINT('Ctrl Pts',(-0.181850551972504,0.0694252034091049,
-0.0254000000000002));
#25055=CARTESIAN_POINT('Ctrl Pts',(-0.183229787629028,0.0636315522952145,
-0.0254000000000002));
#25056=CARTESIAN_POINT('Ctrl Pts',(-0.18542372495759,0.0544156453634958,
-0.0254000000000003));
#25057=CARTESIAN_POINT('Ctrl Pts',(-0.186874660056435,0.045021678959618,
-0.0254000000000002));
#25058=CARTESIAN_POINT('Ctrl Pts',(-0.187601227544073,0.0355338426658405,
-0.0254000000000001));
#25059=CARTESIAN_POINT('Ctrl Pts',(-0.187947943303617,0.0310062765099001,
-0.0254000000000001));
#25060=CARTESIAN_POINT('Ctrl Pts',(-0.188129147364736,0.026457242532671,
-0.0254000000000002));
#25061=CARTESIAN_POINT('Ctrl Pts',(-0.188146660120574,0.0219107093455789,
-0.0254000000000002));
#25062=CARTESIAN_POINT('Ctrl Pts',(-0.188174227502584,0.0147538678781792,
-0.0254000000000002));
#25063=CARTESIAN_POINT('Ctrl Pts',(-0.187797349460741,0.00759407962602553,
-0.0254000000000002));
#25064=CARTESIAN_POINT('Ctrl Pts',(-0.187024335822518,0.000468048982504179,
-0.0254000000000002));
#25065=CARTESIAN_POINT('Ctrl Pts',(-0.186499030634634,-0.00437447989534716,
-0.0254000000000002));
#25066=CARTESIAN_POINT('Ctrl Pts',(-0.185790682000941,-0.00920140104915156,
-0.0254000000000003));
#25067=CARTESIAN_POINT('Ctrl Pts',(-0.184900643419175,-0.0140005797065861,
-0.0254000000000003));
#25068=CARTESIAN_POINT('Ctrl Pts',(-0.184132779193588,-0.0181409817955999,
-0.0254000000000003));
#25069=CARTESIAN_POINT('Ctrl Pts',(-0.183229102993718,-0.0222617381008127,
-0.0254000000000004));
#25070=CARTESIAN_POINT('Ctrl Pts',(-0.182194971678485,-0.0263383737172839,
-0.0254000000000003));
#25071=CARTESIAN_POINT('Ctrl Pts',(-0.179181975057578,-0.0382158685345879,
-0.0254000000000003));
#25072=CARTESIAN_POINT('Ctrl Pts',(-0.175059469051961,-0.0497546103305461,
-0.0254000000000002));
#25073=CARTESIAN_POINT('Ctrl Pts',(-0.169859086925564,-0.0607628510176612,
-0.0254000000000002));
#25074=CARTESIAN_POINT('Ctrl Pts',(-0.167269936719285,-0.0662435999228502,
-0.0254000000000001));
#25075=CARTESIAN_POINT('Ctrl Pts',(-0.164412932388428,-0.0715924281006022,
-0.0254000000000001));
#25076=CARTESIAN_POINT('Ctrl Pts',(-0.161288438287051,-0.0767821423128327,
-0.0254000000000002));
#25077=CARTESIAN_POINT('Ctrl Pts',(-0.158668603425435,-0.0811336289131844,
-0.0254000000000002));
#25078=CARTESIAN_POINT('Ctrl Pts',(-0.155857058035564,-0.0853773956860439,
-0.0254000000000001));
#25079=CARTESIAN_POINT('Ctrl Pts',(-0.152872677055221,-0.0894708909542363,
-0.0254000000000001));
#25080=CARTESIAN_POINT('Ctrl Pts',(-0.148577680288583,-0.0953620787941746,
-0.0254000000000002));
#25081=CARTESIAN_POINT('Ctrl Pts',(-0.143920174645333,-0.100952225610252,
-0.0254000000000002));
#25082=CARTESIAN_POINT('Ctrl Pts',(-0.138904565814662,-0.106196500366509,
-0.0254000000000002));
#25083=CARTESIAN_POINT('Ctrl Pts',(-0.133141847811386,-0.112221945645895,
-0.0254000000000001));
#25084=CARTESIAN_POINT('Ctrl Pts',(-0.126906212836165,-0.117791094215227,
-0.0254000000000001));
#25085=CARTESIAN_POINT('Ctrl Pts',(-0.120262137870373,-0.122877728119754,
-0.0254000000000001));
#25086=CARTESIAN_POINT('Ctrl Pts',(-0.117196150482267,-0.125225015812847,
-0.0254000000000001));
#25087=CARTESIAN_POINT('Ctrl Pts',(-0.114043125364532,-0.127469381869944,
-0.0254));
#25088=CARTESIAN_POINT('Ctrl Pts',(-0.110809234819109,-0.129607334440998,
-0.0254));
#25089=CARTESIAN_POINT('Ctrl Pts',(-0.107698297930514,-0.131664001302767,
-0.0254));
#25090=CARTESIAN_POINT('Ctrl Pts',(-0.104518672572365,-0.133617962067455,
-0.0254000000000002));
#25091=CARTESIAN_POINT('Ctrl Pts',(-0.101282336137666,-0.135464061965196,
-0.0254000000000002));
#25092=CARTESIAN_POINT('Ctrl Pts',(-0.0928811385341354,-0.140256348042283,
-0.0254000000000002));
#25093=CARTESIAN_POINT('Ctrl Pts',(-0.084085973651599,-0.144331678880361,
-0.0254000000000001));
#25094=CARTESIAN_POINT('Ctrl Pts',(-0.075000622341404,-0.147649433262726,
-0.0254000000000001));
#25095=CARTESIAN_POINT('Ctrl Pts',(-0.0691135240229781,-0.149799261659946,
-0.0254000000000002));
#25096=CARTESIAN_POINT('Ctrl Pts',(-0.0631044080958086,-0.151630500595275,
-0.0254));
#25097=CARTESIAN_POINT('Ctrl Pts',(-0.0570016890090982,-0.153126178223591,
-0.0254));
#25098=CARTESIAN_POINT('Ctrl Pts',(-0.0525695195872538,-0.15421243117985,
-0.0254));
#25099=CARTESIAN_POINT('Ctrl Pts',(-0.0480836796866101,-0.155121871124085,
-0.0254000000000002));
#25100=CARTESIAN_POINT('Ctrl Pts',(-0.0435831167051402,-0.155843198108109,
-0.0254000000000002));
#25101=CARTESIAN_POINT('Ctrl Pts',(-0.032940985490312,-0.157548863920228,
-0.0254000000000002));
#25102=CARTESIAN_POINT('Ctrl Pts',(-0.0221883550620207,-0.158214788306086,
-0.0254000000000002));
#25103=CARTESIAN_POINT('Ctrl Pts',(-0.0114741912448819,-0.15776348171624,
-0.0254000000000002));
#25104=CARTESIAN_POINT('Ctrl Pts',(-0.00407369102796414,-0.157451754681536,
-0.0254000000000002));
#25105=CARTESIAN_POINT('Ctrl Pts',(0.00330847097457228,-0.156606036832058,
-0.0254000000000001));
#25106=CARTESIAN_POINT('Ctrl Pts',(0.0106175386826097,-0.155187210724091,
-0.0254000000000001));
#25107=CARTESIAN_POINT('Ctrl Pts',(-0.0685825729128711,0.139614588036676,
-0.476074074893873));
#25108=CARTESIAN_POINT('Ctrl Pts',(-0.11449921200636,0.117059056463457,
-0.472410058024817));
#25109=CARTESIAN_POINT('Ctrl Pts',(-0.181611195120813,0.0235386823327614,
-0.465082024286706));
#25110=CARTESIAN_POINT('Ctrl Pts',(-0.119678168822871,-0.138828443538179,
-0.454089973679538));
#25111=CARTESIAN_POINT('Ctrl Pts',(0.0497528850778061,-0.176238783935,-0.443097923072371));
#25112=CARTESIAN_POINT('Ctrl Pts',(0.174480439215212,-0.0557730335995584,
-0.432105872465203));
#25113=CARTESIAN_POINT('Ctrl Pts',(0.142735182152908,0.114832328488475,
-0.421113821858035));
#25114=CARTESIAN_POINT('Ctrl Pts',(-0.017066041194646,0.182373641719569,
-0.410121771250868));
#25115=CARTESIAN_POINT('Ctrl Pts',(-0.16154811780732,0.0863532198846474,
-0.3991297206437));
#25116=CARTESIAN_POINT('Ctrl Pts',(-0.161124636119803,-0.0871431951720242,
-0.388137670036532));
#25117=CARTESIAN_POINT('Ctrl Pts',(-0.016166963865162,-0.182462532985216,
-0.377145619429364));
#25118=CARTESIAN_POINT('Ctrl Pts',(0.143291190860782,-0.114114530259385,
-0.366153568822197));
#25119=CARTESIAN_POINT('Ctrl Pts',(0.174215754599295,0.0565982325616605,
-0.35516151821503));
#25120=CARTESIAN_POINT('Ctrl Pts',(0.0488656965331514,0.176540319869506,
-0.344169467607861));
#25121=CARTESIAN_POINT('Ctrl Pts',(-0.120317419627598,0.138123660865276,
-0.333177417000694));
#25122=CARTESIAN_POINT('Ctrl Pts',(-0.181574082384246,-0.0241923660424905,
-0.322185366393526));
#25123=CARTESIAN_POINT('Ctrl Pts',(-0.0799559507003814,-0.164807298147092,
-0.311193315786359));
#25124=CARTESIAN_POINT('Ctrl Pts',(0.0933838621769322,-0.157587648721984,
-0.300201265179191));
#25125=CARTESIAN_POINT('Ctrl Pts',(0.182956936375875,-0.00900941659901149,
-0.289209214572024));
#25126=CARTESIAN_POINT('Ctrl Pts',(0.108414826916839,0.14765037535385,-0.278217163964856));
#25127=CARTESIAN_POINT('Ctrl Pts',(-0.0633770392495001,0.17186553164345,
-0.267225113357688));
#25128=CARTESIAN_POINT('Ctrl Pts',(-0.178318731760777,0.0419146652942395,
-0.25623306275052));
#25129=CARTESIAN_POINT('Ctrl Pts',(-0.133305789961508,-0.125634293193532,
-0.245241012143353));
#25130=CARTESIAN_POINT('Ctrl Pts',(0.031284490132526,-0.180487370051941,
-0.234248961536185));
#25131=CARTESIAN_POINT('Ctrl Pts',(0.167812098115434,-0.0734405049249859,
-0.223256910929018));
#25132=CARTESIAN_POINT('Ctrl Pts',(0.15380969315891,0.0994836089306307,
-0.21226486032185));
#25133=CARTESIAN_POINT('Ctrl Pts',(0.00183761696418741,0.183169418595726,
-0.201272809714682));
#25134=CARTESIAN_POINT('Ctrl Pts',(-0.151782791833885,0.102549420661736,
-0.190280759107515));
#25135=CARTESIAN_POINT('Ctrl Pts',(-0.169251783292637,-0.0700589167820705,
-0.179288708500347));
#25136=CARTESIAN_POINT('Ctrl Pts',(-0.0348991934490358,-0.179823450787922,
-0.168296657893179));
#25137=CARTESIAN_POINT('Ctrl Pts',(0.130758243427182,-0.128283368419821,
-0.157304607286012));
#25138=CARTESIAN_POINT('Ctrl Pts',(0.179124036706147,0.0383284300983071,
-0.146312556678844));
#25139=CARTESIAN_POINT('Ctrl Pts',(0.0668118623371123,0.17055986176609,
-0.135320506071676));
#25140=CARTESIAN_POINT('Ctrl Pts',(-0.105429739997846,0.149794915093888,
-0.124328455464509));
#25141=CARTESIAN_POINT('Ctrl Pts',(-0.183102754328823,-0.00533537128298008,
-0.113336404857341));
#25142=CARTESIAN_POINT('Ctrl Pts',(-0.0965231054289514,-0.155685461973447,
-0.102344354250173));
#25143=CARTESIAN_POINT('Ctrl Pts',(0.0766264864264418,-0.166372403162464,
-0.091352303643006));
#25144=CARTESIAN_POINT('Ctrl Pts',(0.181065301238179,-0.0278415620581252,
-0.0803602530358381));
#25145=CARTESIAN_POINT('Ctrl Pts',(0.123039270360697,0.135703326763709,
-0.0693682024286707));
#25146=CARTESIAN_POINT('Ctrl Pts',(-0.0452659821533855,0.177444214884968,
-0.058376151821503));
#25147=CARTESIAN_POINT('Ctrl Pts',(-0.173137980058957,0.0601617876158408,
-0.0473841012143354));
#25148=CARTESIAN_POINT('Ctrl Pts',(-0.145363928230217,-0.111382333108322,
-0.0363920506071676));
#25149=CARTESIAN_POINT('Ctrl Pts',(-0.0404206461299352,-0.158679121552366,
-0.029064016869056));
#25150=CARTESIAN_POINT('Ctrl Pts',(0.0106175386826097,-0.155187210724091,
-0.0254000000000001));
#25151=CARTESIAN_POINT('Ctrl Pts',(-0.0744392439309313,0.151537102412036,
-0.468404938818138));
#25152=CARTESIAN_POINT('Ctrl Pts',(-0.124276976066047,0.12705542076233,
-0.464740921949082));
#25153=CARTESIAN_POINT('Ctrl Pts',(-0.197120047848906,0.0255487894600746,
-0.45741288821097));
#25154=CARTESIAN_POINT('Ctrl Pts',(-0.129898194597202,-0.150683824391059,
-0.446420837603803));
#25155=CARTESIAN_POINT('Ctrl Pts',(0.0540015778247265,-0.191288854737121,
-0.435428786996635));
#25156=CARTESIAN_POINT('Ctrl Pts',(0.189380354575173,-0.0605358223897492,
-0.424436736389467));
#25157=CARTESIAN_POINT('Ctrl Pts',(0.154924182493192,0.124638539332289,
-0.413444685782299));
#25158=CARTESIAN_POINT('Ctrl Pts',(-0.0185234112613053,0.197947604266499,
-0.402452635175133));
#25159=CARTESIAN_POINT('Ctrl Pts',(-0.175343665851082,0.0937274314187808,
-0.391460584567963));
#25160=CARTESIAN_POINT('Ctrl Pts',(-0.174884020560764,-0.0945848673623276,
-0.380468533960798));
#25161=CARTESIAN_POINT('Ctrl Pts',(-0.0175475564078102,-0.1980440864824,
-0.369476483353628));
#25162=CARTESIAN_POINT('Ctrl Pts',(0.155527672068972,-0.123859444072385,
-0.358484432746461));
#25163=CARTESIAN_POINT('Ctrl Pts',(0.189093066976413,0.061431489965672,
-0.347492382139294));
#25164=CARTESIAN_POINT('Ctrl Pts',(0.0530386270096244,0.191616140606247,
-0.336500331532126));
#25165=CARTESIAN_POINT('Ctrl Pts',(-0.130592034804196,0.149918856162568,
-0.325508280924959));
#25166=CARTESIAN_POINT('Ctrl Pts',(-0.197079765836539,-0.0262582950830843,
-0.314516230317791));
#25167=CARTESIAN_POINT('Ctrl Pts',(-0.0867838616302223,-0.178881166852035,
-0.303524179710623));
#25168=CARTESIAN_POINT('Ctrl Pts',(0.101358461786384,-0.171044988916071,
-0.292532129103456));
#25169=CARTESIAN_POINT('Ctrl Pts',(0.198580709899027,-0.0097787839009954,
-0.281540078496288));
#25170=CARTESIAN_POINT('Ctrl Pts',(0.117673009393291,0.160259113075592,
-0.27054802788912));
#25171=CARTESIAN_POINT('Ctrl Pts',(-0.0687891789989752,0.186542144599608,
-0.259555977281953));
#25172=CARTESIAN_POINT('Ctrl Pts',(-0.193546421593985,0.0454940061535037,
-0.248563926674785));
#25173=CARTESIAN_POINT('Ctrl Pts',(-0.14468955880318,-0.13636294761068,
-0.237571876067617));
#25174=CARTESIAN_POINT('Ctrl Pts',(0.0339560575423216,-0.195900252718971,
-0.226579825460449));
#25175=CARTESIAN_POINT('Ctrl Pts',(0.182142564439017,-0.0797120234533494,
-0.215587774853282));
#25176=CARTESIAN_POINT('Ctrl Pts',(0.166944411411096,0.107979101946565,
-0.204595724246114));
#25177=CARTESIAN_POINT('Ctrl Pts',(0.00199454193155687,0.198811337230763,
-0.193603673638947));
#25178=CARTESIAN_POINT('Ctrl Pts',(-0.164744421009028,0.111306721451129,
-0.182611623031779));
#25179=CARTESIAN_POINT('Ctrl Pts',(-0.183705192837717,-0.0760416615238799,
-0.171619572424612));
#25180=CARTESIAN_POINT('Ctrl Pts',(-0.037879441727069,-0.195179637467229,
-0.160627521817444));
#25181=CARTESIAN_POINT('Ctrl Pts',(0.141924462221939,-0.13923824301862,
-0.149635471210276));
#25182=CARTESIAN_POINT('Ctrl Pts',(0.194420496285574,0.0416015211503103,
-0.138643420603109));
#25183=CARTESIAN_POINT('Ctrl Pts',(0.0725173219195277,0.185124975858833,
-0.127651369995941));
#25184=CARTESIAN_POINT('Ctrl Pts',(-0.114433008269386,0.162586787731822,
-0.116659319388773));
#25185=CARTESIAN_POINT('Ctrl Pts',(-0.198738980108323,-0.00579099015285377,
-0.105667268781606));
#25186=CARTESIAN_POINT('Ctrl Pts',(-0.104765783563193,-0.168980363204866,
-0.0946752181744379));
#25187=CARTESIAN_POINT('Ctrl Pts',(0.0831700747347963,-0.180579925429739,
-0.0836831675672704));
#25188=CARTESIAN_POINT('Ctrl Pts',(0.19652753686304,-0.0302191175022836,
-0.0726911169601027));
#25189=CARTESIAN_POINT('Ctrl Pts',(0.133546320449358,0.147291835435162,
-0.0616990663529351));
#25190=CARTESIAN_POINT('Ctrl Pts',(-0.0491315117554692,0.192597224556383,
-0.0507070157457675));
#25191=CARTESIAN_POINT('Ctrl Pts',(-0.187923254901664,0.0652993580358375,
-0.0397149651385998));
#25192=CARTESIAN_POINT('Ctrl Pts',(-0.157777412726036,-0.120893928467513,
-0.0287229145314321));
#25193=CARTESIAN_POINT('Ctrl Pts',(-0.043872403867593,-0.172229669058767,
-0.0213948807933204));
#25194=CARTESIAN_POINT('Ctrl Pts',(0.0115242330284832,-0.168439563338159,
-0.0177308639242646));
#25195=CARTESIAN_POINT('Ctrl Pts',(-0.0802959149489916,0.163459616787395,
-0.460735802742402));
#25196=CARTESIAN_POINT('Ctrl Pts',(-0.134054740125735,0.137051785061202,
-0.457071785873346));
#25197=CARTESIAN_POINT('Ctrl Pts',(-0.212628900576999,0.0275588965873877,
-0.449743752135234));
#25198=CARTESIAN_POINT('Ctrl Pts',(-0.140118220371533,-0.162539205243939,
-0.438751701528067));
#25199=CARTESIAN_POINT('Ctrl Pts',(0.0582502705716468,-0.206338925539242,
-0.427759650920899));
#25200=CARTESIAN_POINT('Ctrl Pts',(0.204280269935135,-0.06529861117994,
-0.416767600313732));
#25201=CARTESIAN_POINT('Ctrl Pts',(0.167113182833476,0.134444750176102,
-0.405775549706564));
#25202=CARTESIAN_POINT('Ctrl Pts',(-0.0199807813279645,0.213521566813429,
-0.394783499099397));
#25203=CARTESIAN_POINT('Ctrl Pts',(-0.189139213894845,0.101101642952914,
-0.383791448492229));
#25204=CARTESIAN_POINT('Ctrl Pts',(-0.188643405001724,-0.102026539552631,
-0.372799397885061));
#25205=CARTESIAN_POINT('Ctrl Pts',(-0.0189281489504585,-0.213625639979584,
-0.361807347277894));
#25206=CARTESIAN_POINT('Ctrl Pts',(0.167764153277162,-0.133604357885385,
-0.350815296670725));
#25207=CARTESIAN_POINT('Ctrl Pts',(0.203970379353531,0.0662647473696836,
-0.339823246063558));
#25208=CARTESIAN_POINT('Ctrl Pts',(0.0572115574860978,0.206691961342987,
-0.328831195456391));
#25209=CARTESIAN_POINT('Ctrl Pts',(-0.140866649980795,0.16171405145986,
-0.317839144849223));
#25210=CARTESIAN_POINT('Ctrl Pts',(-0.212585449288831,-0.0283242241236782,
-0.306847094242055));
#25211=CARTESIAN_POINT('Ctrl Pts',(-0.0936117725600636,-0.192955035556977,
-0.295855043634888));
#25212=CARTESIAN_POINT('Ctrl Pts',(0.109333061395836,-0.18450232911016,
-0.28486299302772));
#25213=CARTESIAN_POINT('Ctrl Pts',(0.214204483422178,-0.0105481512029789,
-0.273870942420553));
#25214=CARTESIAN_POINT('Ctrl Pts',(0.126931191869743,0.172867850797333,
-0.262878891813384));
#25215=CARTESIAN_POINT('Ctrl Pts',(-0.07420131874845,0.201218757555768,
-0.251886841206217));
#25216=CARTESIAN_POINT('Ctrl Pts',(-0.208774111427194,0.0490733470127675,
-0.240894790599049));
#25217=CARTESIAN_POINT('Ctrl Pts',(-0.156073327644852,-0.147091602027827,
-0.229902739991882));
#25218=CARTESIAN_POINT('Ctrl Pts',(0.0366276249521169,-0.211313135386002,
-0.218910689384714));
#25219=CARTESIAN_POINT('Ctrl Pts',(0.1964730307626,-0.0859835419817126,
-0.207918638777546));
#25220=CARTESIAN_POINT('Ctrl Pts',(0.180079129663282,0.116474594962498,
-0.196926588170379));
#25221=CARTESIAN_POINT('Ctrl Pts',(0.00215146689892645,0.214453255865799,
-0.185934537563211));
#25222=CARTESIAN_POINT('Ctrl Pts',(-0.17770605018417,0.120064022240522,
-0.174942486956044));
#25223=CARTESIAN_POINT('Ctrl Pts',(-0.198158602382797,-0.0820244062656893,
-0.163950436348876));
#25224=CARTESIAN_POINT('Ctrl Pts',(-0.0408596900051022,-0.210535824146536,
-0.152958385741708));
#25225=CARTESIAN_POINT('Ctrl Pts',(0.153090681016695,-0.15019311761742,
-0.141966335134541));
#25226=CARTESIAN_POINT('Ctrl Pts',(0.209716955865002,0.0448746122023138,
-0.130974284527373));
#25227=CARTESIAN_POINT('Ctrl Pts',(0.0782227815019429,0.199690089951577,
-0.119982233920205));
#25228=CARTESIAN_POINT('Ctrl Pts',(-0.123436276540926,0.175378660369755,
-0.108990183313038));
#25229=CARTESIAN_POINT('Ctrl Pts',(-0.214375205887822,-0.0062466090227276,
-0.0979981327058702));
#25230=CARTESIAN_POINT('Ctrl Pts',(-0.113008461697435,-0.182275264436286,
-0.0870060820987024));
#25231=CARTESIAN_POINT('Ctrl Pts',(0.0897136630431509,-0.194787447697015,
-0.076014031491535));
#25232=CARTESIAN_POINT('Ctrl Pts',(0.211989772487901,-0.0325966729464418,
-0.0650219808843671));
#25233=CARTESIAN_POINT('Ctrl Pts',(0.14405337053802,0.158880344106616,-0.0540299302771997));
#25234=CARTESIAN_POINT('Ctrl Pts',(-0.0529970413575529,0.207750234227798,
-0.0430378796700319));
#25235=CARTESIAN_POINT('Ctrl Pts',(-0.202708529744371,0.0704369284558339,
-0.0320458290628643));
#25236=CARTESIAN_POINT('Ctrl Pts',(-0.170190897221856,-0.130405523826704,
-0.0210537784556966));
#25237=CARTESIAN_POINT('Ctrl Pts',(-0.0473241616052508,-0.185780216565167,
-0.0137257447175849));
#25238=CARTESIAN_POINT('Ctrl Pts',(0.0124309273743567,-0.181691915952227,
-0.010061727848529));
#25239=CARTESIAN_POINT('Ctrl Pts',(-0.0861525859670518,0.175382131162755,
-0.453066666666667));
#25240=CARTESIAN_POINT('Ctrl Pts',(-0.143832504185423,0.147048149360075,
-0.449402649797611));
#25241=CARTESIAN_POINT('Ctrl Pts',(-0.228137753305091,0.0295690037147008,
-0.442074616059499));
#25242=CARTESIAN_POINT('Ctrl Pts',(-0.150338246145864,-0.174394586096819,
-0.431082565452331));
#25243=CARTESIAN_POINT('Ctrl Pts',(0.0624989633185675,-0.221388996341363,
-0.420090514845164));
#25244=CARTESIAN_POINT('Ctrl Pts',(0.219180185295097,-0.0700613999701309,
-0.409098464237996));
#25245=CARTESIAN_POINT('Ctrl Pts',(0.17930218317376,0.144250961019916,-0.398106413630828));
#25246=CARTESIAN_POINT('Ctrl Pts',(-0.0214381513946237,0.229095529360358,
-0.387114363023661));
#25247=CARTESIAN_POINT('Ctrl Pts',(-0.202934761938607,0.108475854487047,
-0.376122312416493));
#25248=CARTESIAN_POINT('Ctrl Pts',(-0.202402789442685,-0.109468211742934,
-0.365130261809326));
#25249=CARTESIAN_POINT('Ctrl Pts',(-0.0203087414931069,-0.229207193476768,
-0.354138211202158));
#25250=CARTESIAN_POINT('Ctrl Pts',(0.180000634485353,-0.143349271698386,
-0.34314616059499));
#25251=CARTESIAN_POINT('Ctrl Pts',(0.218847691730649,0.0710980047736953,
-0.332154109987823));
#25252=CARTESIAN_POINT('Ctrl Pts',(0.0613844879625708,0.221767782079727,
-0.321162059380655));
#25253=CARTESIAN_POINT('Ctrl Pts',(-0.151141265157393,0.173509246757153,
-0.310170008773488));
#25254=CARTESIAN_POINT('Ctrl Pts',(-0.228091132741123,-0.030390153164272,
-0.29917795816632));
#25255=CARTESIAN_POINT('Ctrl Pts',(-0.100439683489904,-0.20702890426192,
-0.288185907559152));
#25256=CARTESIAN_POINT('Ctrl Pts',(0.117307661005287,-0.197959669304247,
-0.277193856951985));
#25257=CARTESIAN_POINT('Ctrl Pts',(0.22982825694533,-0.011317518504963,
-0.266201806344817));
#25258=CARTESIAN_POINT('Ctrl Pts',(0.136189374346194,0.185476588519076,
-0.255209755737649));
#25259=CARTESIAN_POINT('Ctrl Pts',(-0.0796134584979247,0.215895370511926,
-0.244217705130482));
#25260=CARTESIAN_POINT('Ctrl Pts',(-0.224001801260403,0.0526526878720317,
-0.233225654523314));
#25261=CARTESIAN_POINT('Ctrl Pts',(-0.167457096486523,-0.157820256444976,
-0.222233603916146));
#25262=CARTESIAN_POINT('Ctrl Pts',(0.0392991923619123,-0.226726018053033,
-0.211241553308979));
#25263=CARTESIAN_POINT('Ctrl Pts',(0.210803497086183,-0.0922550605100761,
-0.200249502701811));
#25264=CARTESIAN_POINT('Ctrl Pts',(0.193213847915468,0.124970087978432,
-0.189257452094643));
#25265=CARTESIAN_POINT('Ctrl Pts',(0.00230839186629608,0.230095174500836,
-0.178265401487476));
#25266=CARTESIAN_POINT('Ctrl Pts',(-0.190667679359313,0.128821323029915,
-0.167273350880308));
#25267=CARTESIAN_POINT('Ctrl Pts',(-0.212612011927877,-0.0880071510074988,
-0.15628130027314));
#25268=CARTESIAN_POINT('Ctrl Pts',(-0.0438399382831356,-0.225892010825843,
-0.145289249665973));
#25269=CARTESIAN_POINT('Ctrl Pts',(0.164256899811452,-0.16114799221622,
-0.134297199058805));
#25270=CARTESIAN_POINT('Ctrl Pts',(0.22501341544443,0.0481477032543172,
-0.123305148451638));
#25271=CARTESIAN_POINT('Ctrl Pts',(0.0839282410843581,0.21425520404432,
-0.11231309784447));
#25272=CARTESIAN_POINT('Ctrl Pts',(-0.132439544812465,0.188170533007688,
-0.101321047237302));
#25273=CARTESIAN_POINT('Ctrl Pts',(-0.230011431667322,-0.00670222789260128,
-0.0903289966301345));
#25274=CARTESIAN_POINT('Ctrl Pts',(-0.121251139831676,-0.195570165667705,
-0.079336946022967));
#25275=CARTESIAN_POINT('Ctrl Pts',(0.0962572513515054,-0.208994969964291,
-0.0683448954157993));
#25276=CARTESIAN_POINT('Ctrl Pts',(0.227452008112762,-0.0349742283906001,
-0.0573528448086317));
#25277=CARTESIAN_POINT('Ctrl Pts',(0.154560420626681,0.170468852778069,
-0.0463607942014641));
#25278=CARTESIAN_POINT('Ctrl Pts',(-0.0568625709596362,0.222903243899213,
-0.0353687435942964));
#25279=CARTESIAN_POINT('Ctrl Pts',(-0.217493804587078,0.0755744988758305,
-0.0243766929871288));
#25280=CARTESIAN_POINT('Ctrl Pts',(-0.182604381717675,-0.139917119185895,
-0.0133846423799611));
#25281=CARTESIAN_POINT('Ctrl Pts',(-0.0507759193429087,-0.199330764071568,
-0.00605660864184936));
#25282=CARTESIAN_POINT('Ctrl Pts',(0.0133376217202303,-0.194944268566296,
-0.0023925917727935));
#25283=CARTESIAN_POINT('Ctrl Pts',(-0.195698342875023,-3.28562868159645E-5,
-0.0906536358790898));
#25284=CARTESIAN_POINT('Ctrl Pts',(-0.195702885553977,-0.00192275150872445,
-0.0905454227961047));
#25285=CARTESIAN_POINT('Ctrl Pts',(-0.195677808282155,-0.0038125242527969,
-0.0904372097131196));
#25286=CARTESIAN_POINT('Ctrl Pts',(-0.195622735218905,-0.00570142403840418,
-0.0903289966301345));
#25287=CARTESIAN_POINT('Ctrl Pts',(-0.19375800105544,-0.0696582071509693,
-0.0866649797610786));
#25288=CARTESIAN_POINT('Ctrl Pts',(-0.157504570443558,-0.132614186409337,
-0.0830009628920228));
#25289=CARTESIAN_POINT('Ctrl Pts',(-0.103126456607088,-0.166329643421285,
-0.079336946022967));
#25290=CARTESIAN_POINT('Ctrl Pts',(-0.0487483427706158,-0.200045100433234,
-0.0756729291539111));
#25291=CARTESIAN_POINT('Ctrl Pts',(0.0237544542904457,-0.204520035198762,
-0.0720089122848551));
#25292=CARTESIAN_POINT('Ctrl Pts',(0.0818716456145191,-0.177754045652577,
-0.0683448954157992));
#25293=CARTESIAN_POINT('Ctrl Pts',(0.139988836938592,-0.150988056106393,
-0.0646808785467433));
#25294=CARTESIAN_POINT('Ctrl Pts',(0.183720422525678,-0.0929811422484953,
-0.0610168616776875));
#25295=CARTESIAN_POINT('Ctrl Pts',(0.193437617404873,-0.0297371717914351,
-0.0573528448086316));
#25296=CARTESIAN_POINT('Ctrl Pts',(0.203154812284068,0.0335067986656242,
-0.0536888279395758));
#25297=CARTESIAN_POINT('Ctrl Pts',(0.178857616455375,0.101987825721846,
-0.0500248110705199));
#25298=CARTESIAN_POINT('Ctrl Pts',(0.131471853276642,0.144967404436815,
-0.0463607942014641));
#25299=CARTESIAN_POINT('Ctrl Pts',(0.084086090097909,0.187946983151784,
-0.0426967773324082));
#25300=CARTESIAN_POINT('Ctrl Pts',(0.0136117595691364,0.205425113525499,
-0.0390327604633523));
#25301=CARTESIAN_POINT('Ctrl Pts',(-0.0483972779664903,0.189609387875126,
-0.0353687435942964));
#25302=CARTESIAN_POINT('Ctrl Pts',(-0.104633572522728,0.175266030170468,
-0.0320458290628643));
#25303=CARTESIAN_POINT('Ctrl Pts',(-0.153907363890767,0.133539263657296,
-0.0287229145314322));
#25304=CARTESIAN_POINT('Ctrl Pts',(-0.178226250896966,0.0807893643570689,
-0.0254000000000001));
#25305=CARTESIAN_POINT('',(-0.0903606778650201,-0.126612599672284,-0.453066666666667));
#25306=CARTESIAN_POINT('Ctrl Pts',(-0.0905470291188205,-0.126755563903434,
-0.453066666666667));
#25307=CARTESIAN_POINT('Ctrl Pts',(-0.0947991957642303,-0.124487575468212,
-0.453066666666667));
#25308=CARTESIAN_POINT('Ctrl Pts',(-0.0989294677700178,-0.122016794807246,
-0.453066666666667));
#25309=CARTESIAN_POINT('Ctrl Pts',(-0.10292135951426,-0.119346893969649,
-0.453066666666667));
#25310=CARTESIAN_POINT('Ctrl Pts',(-0.108133628568249,-0.115860766989102,
-0.453066666666667));
#25311=CARTESIAN_POINT('Ctrl Pts',(-0.113110147998552,-0.112035408131854,
-0.453066666666667));
#25312=CARTESIAN_POINT('Ctrl Pts',(-0.117841914883643,-0.107907652239557,
-0.453066666666667));
#25313=CARTESIAN_POINT('Ctrl Pts',(-0.122114349501896,-0.104180594758025,
-0.453066666666667));
#25314=CARTESIAN_POINT('Ctrl Pts',(-0.126190272687336,-0.100202764591398,
-0.453066666666667));
#25315=CARTESIAN_POINT('Ctrl Pts',(-0.130041327864726,-0.0960214698833582,
-0.453066666666667));
#25316=CARTESIAN_POINT('Ctrl Pts',(-0.135935559478366,-0.089621790232241,
-0.453066666666667));
#25317=CARTESIAN_POINT('Ctrl Pts',(-0.141313195335496,-0.0827394474627572,
-0.453066666666667));
#25318=CARTESIAN_POINT('Ctrl Pts',(-0.146148572761508,-0.0754634735042225,
-0.453066666666667));
#25319=CARTESIAN_POINT('Ctrl Pts',(-0.149168330159111,-0.0709195311704024,
-0.453066666666667));
#25320=CARTESIAN_POINT('Ctrl Pts',(-0.151978671030338,-0.0662164416771034,
-0.453066666666667));
#25321=CARTESIAN_POINT('Ctrl Pts',(-0.154556741894587,-0.0614028695358839,
-0.453066666666667));
#25322=CARTESIAN_POINT('Ctrl Pts',(-0.160075954266155,-0.0510978281649633,
-0.453066666666667));
#25323=CARTESIAN_POINT('Ctrl Pts',(-0.164547838171259,-0.040270898794287,
-0.453066666666667));
#25324=CARTESIAN_POINT('Ctrl Pts',(-0.167909402584567,-0.0291166800107643,
-0.453066666666667));
#25325=CARTESIAN_POINT('Ctrl Pts',(-0.169458518128482,-0.0239764620725413,
-0.453066666666667));
#25326=CARTESIAN_POINT('Ctrl Pts',(-0.17077135633224,-0.0187661737549059,
-0.453066666666667));
#25327=CARTESIAN_POINT('Ctrl Pts',(-0.171838785035581,-0.0135026857692308,
-0.453066666666667));
#25328=CARTESIAN_POINT('Ctrl Pts',(-0.172761838697209,-0.00895111071517557,
-0.453066666666667));
#25329=CARTESIAN_POINT('Ctrl Pts',(-0.173501415363079,-0.00435555596891192,
-0.453066666666667));
#25330=CARTESIAN_POINT('Ctrl Pts',(-0.174048163489164,0.000245370197640356,
-0.453066666666667));
#25331=CARTESIAN_POINT('Ctrl Pts',(-0.174928992407005,0.00765761108701054,
-0.453066666666667));
#25332=CARTESIAN_POINT('Ctrl Pts',(-0.175313137595295,0.0150962164885127,
-0.453066666666667));
#25333=CARTESIAN_POINT('Ctrl Pts',(-0.17518323296547,0.0225143573359635,
-0.453066666666667));
#25334=CARTESIAN_POINT('Ctrl Pts',(-0.175047559449211,0.0302619276437026,
-0.453066666666667));
#25335=CARTESIAN_POINT('Ctrl Pts',(-0.174351423432551,0.0379873668160185,
-0.453066666666667));
#25336=CARTESIAN_POINT('Ctrl Pts',(-0.173130401268424,0.0456510136887945,
-0.453066666666667));
#25337=CARTESIAN_POINT('Ctrl Pts',(-0.172378019222284,0.0503732787585368,
-0.453066666666667));
#25338=CARTESIAN_POINT('Ctrl Pts',(-0.171426132330918,0.0550721261644083,
-0.453066666666667));
#25339=CARTESIAN_POINT('Ctrl Pts',(-0.170281162641598,0.0597383409928608,
-0.453066666666667));
#25340=CARTESIAN_POINT('Ctrl Pts',(-0.169381700085032,0.0634040149039102,
-0.453066666666667));
#25341=CARTESIAN_POINT('Ctrl Pts',(-0.168364960525766,0.0670413292940973,
-0.453066666666667));
#25342=CARTESIAN_POINT('Ctrl Pts',(-0.167236908480682,0.0706411471149374,
-0.453066666666667));
#25343=CARTESIAN_POINT('Ctrl Pts',(-0.163878286349993,0.0813591169570331,
-0.453066666666667));
#25344=CARTESIAN_POINT('Ctrl Pts',(-0.159532509087918,0.0917579355296217,
-0.453066666666667));
#25345=CARTESIAN_POINT('Ctrl Pts',(-0.154300403897806,0.101723195040055,
-0.453066666666667));
#25346=CARTESIAN_POINT('Ctrl Pts',(-0.150458279880649,0.109041045410227,
-0.453066666666667));
#25347=CARTESIAN_POINT('Ctrl Pts',(-0.146137323639187,0.11612533476953,
-0.453066666666667));
#25348=CARTESIAN_POINT('Ctrl Pts',(-0.141365363239444,0.122928507327059,
-0.453066666666667));
#25349=CARTESIAN_POINT('Ctrl Pts',(-0.139474935210954,0.12562360682665,
-0.453066666666667));
#25350=CARTESIAN_POINT('Ctrl Pts',(-0.137514595596603,0.128272882481353,
-0.453066666666667));
#25351=CARTESIAN_POINT('Ctrl Pts',(-0.13549208476146,0.130866201634327,
-0.453066666666667));
#25352=CARTESIAN_POINT('Ctrl Pts',(-0.127604957338041,0.140979293862904,
-0.453066666666667));
#25353=CARTESIAN_POINT('Ctrl Pts',(-0.118753988352663,0.150274988313495,
-0.453066666666667));
#25354=CARTESIAN_POINT('Ctrl Pts',(-0.109058348041544,0.1585911082717,-0.453066666666667));
#25355=CARTESIAN_POINT('Ctrl Pts',(-0.101876675688201,0.164750954024479,
-0.453066666666667));
#25356=CARTESIAN_POINT('Ctrl Pts',(-0.0942303837916874,0.17037340113684,
-0.453066666666667));
#25357=CARTESIAN_POINT('Ctrl Pts',(-0.0861525859670518,0.175382131162755,
-0.453066666666667));
#25358=CARTESIAN_POINT('Ctrl Pts',(-0.0905470291188203,-0.126755563903435,
-0.453066666666667));
#25359=CARTESIAN_POINT('Ctrl Pts',(-0.0527502457699392,-0.153392327621369,
-0.449743752135235));
#25360=CARTESIAN_POINT('Ctrl Pts',(0.0536233967596413,-0.172500523394585,
-0.442756820734747));
#25361=CARTESIAN_POINT('Ctrl Pts',(0.174480439215212,-0.0557730335995584,
-0.432105872465203));
#25362=CARTESIAN_POINT('Ctrl Pts',(0.142735182152908,0.114832328488475,
-0.421113821858035));
#25363=CARTESIAN_POINT('Ctrl Pts',(-0.017066041194646,0.182373641719569,
-0.410121771250868));
#25364=CARTESIAN_POINT('Ctrl Pts',(-0.137347945518334,0.102436258045122,
-0.400970845333621));
#25365=CARTESIAN_POINT('Ctrl Pts',(-0.155309689873578,0.0255484863100586,
-0.395483936285431));
#25366=CARTESIAN_POINT('Ctrl Pts',(-0.155306872404023,2.87756186839044E-6,
-0.393661044106296));
#25367=CARTESIAN_POINT('Origin',(-2.59090492670967E-17,0.,-0.453066666666667));
#25368=CARTESIAN_POINT('',(-0.1954,-2.39295984553393E-17,-0.453066666666667));
#25369=CARTESIAN_POINT('Origin',(0.,0.,-0.453066666666667));
#25370=CARTESIAN_POINT('Origin',(0.,0.,-0.453066666666667));
#25371=CARTESIAN_POINT('',(0.0903606778650194,-0.126612599672285,-0.453066666666667));
#25372=CARTESIAN_POINT('Ctrl Pts',(0.0863544310469494,0.175597323663767,
-0.453066666666667));
#25373=CARTESIAN_POINT('Ctrl Pts',(0.0914440695611803,0.172479495245472,
-0.453066666666667));
#25374=CARTESIAN_POINT('Ctrl Pts',(0.096371458315283,0.169121306427088,
-0.453066666666667));
#25375=CARTESIAN_POINT('Ctrl Pts',(0.10111644025993,0.165522169603453,-0.453066666666667));
#25376=CARTESIAN_POINT('Ctrl Pts',(0.108664242830105,0.159797053157331,
-0.453066666666667));
#25377=CARTESIAN_POINT('Ctrl Pts',(0.115751223714214,0.15346251089447,-0.453066666666667));
#25378=CARTESIAN_POINT('Ctrl Pts',(0.122338307079031,0.146595406424471,
-0.453066666666667));
#25379=CARTESIAN_POINT('Ctrl Pts',(0.125481640567847,0.143318447828952,
-0.453066666666667));
#25380=CARTESIAN_POINT('Ctrl Pts',(0.128510764277807,0.139919788637431,
-0.453066666666667));
#25381=CARTESIAN_POINT('Ctrl Pts',(0.131411861578166,0.136419098604737,
-0.453066666666667));
#25382=CARTESIAN_POINT('Ctrl Pts',(0.135978580737029,0.130908539465763,
-0.453066666666667));
#25383=CARTESIAN_POINT('Ctrl Pts',(0.140234769092733,0.125138834436613,
-0.453066666666667));
#25384=CARTESIAN_POINT('Ctrl Pts',(0.144163533941065,0.119143612028972,
-0.453066666666667));
#25385=CARTESIAN_POINT('Ctrl Pts',(0.146833444162397,0.115069378471289,
-0.453066666666667));
#25386=CARTESIAN_POINT('Ctrl Pts',(0.149352043837122,0.110890938917105,
-0.453066666666667));
#25387=CARTESIAN_POINT('Ctrl Pts',(0.151712670729972,0.106618527140408,
-0.453066666666667));
#25388=CARTESIAN_POINT('Ctrl Pts',(0.153749069602213,0.102932923731346,
-0.453066666666667));
#25389=CARTESIAN_POINT('Ctrl Pts',(0.155668099628493,0.0991762472086667,
-0.453066666666667));
#25390=CARTESIAN_POINT('Ctrl Pts',(0.157458355919879,0.0953708013500012,
-0.453066666666667));
#25391=CARTESIAN_POINT('Ctrl Pts',(0.162674643606049,0.0842828356389133,
-0.453066666666667));
#25392=CARTESIAN_POINT('Ctrl Pts',(0.166818779325598,0.0727518602714819,
-0.453066666666667));
#25393=CARTESIAN_POINT('Ctrl Pts',(0.169793416329498,0.0609460732476128,
-0.453066666666667));
#25394=CARTESIAN_POINT('Ctrl Pts',(0.171274420410269,0.0550682405116701,
-0.453066666666667));
#25395=CARTESIAN_POINT('Ctrl Pts',(0.172464744273862,0.0491221862213701,
-0.453066666666667));
#25396=CARTESIAN_POINT('Ctrl Pts',(0.173347398641795,0.0431291460428445,
-0.453066666666667));
#25397=CARTESIAN_POINT('Ctrl Pts',(0.17408748866872,0.038104088185292,-0.453066666666667));
#25398=CARTESIAN_POINT('Ctrl Pts',(0.174611083947877,0.0330404757442079,
-0.453066666666667));
#25399=CARTESIAN_POINT('Ctrl Pts',(0.174905738682316,0.0279831639491109,
-0.453066666666667));
#25400=CARTESIAN_POINT('Ctrl Pts',(0.175329793223554,0.0207048962598366,
-0.453066666666667));
#25401=CARTESIAN_POINT('Ctrl Pts',(0.175282645291204,0.0134289205807883,
-0.453066666666667));
#25402=CARTESIAN_POINT('Ctrl Pts',(0.17473922538412,0.00619266267667447,
-0.453066666666667));
#25403=CARTESIAN_POINT('Ctrl Pts',(0.174114861056575,-0.00212146281144542,
-0.453066666666667));
#25404=CARTESIAN_POINT('Ctrl Pts',(0.172835412310392,-0.0103834978381202,
-0.453066666666667));
#25405=CARTESIAN_POINT('Ctrl Pts',(0.170934029955228,-0.0185322403951933,
-0.453066666666667));
#25406=CARTESIAN_POINT('Ctrl Pts',(0.170056634189217,-0.0222924899833254,
-0.453066666666667));
#25407=CARTESIAN_POINT('Ctrl Pts',(0.169046648886972,-0.026028521993633,
-0.453066666666667));
#25408=CARTESIAN_POINT('Ctrl Pts',(0.167906623664754,-0.0297337195488689,
-0.453066666666667));
#25409=CARTESIAN_POINT('Ctrl Pts',(0.166809883321851,-0.0332982368578347,
-0.453066666666667));
#25410=CARTESIAN_POINT('Ctrl Pts',(0.165594849559875,-0.03682704705354,
-0.453066666666667));
#25411=CARTESIAN_POINT('Ctrl Pts',(0.164267500928256,-0.040308558913606,
-0.453066666666667));
#25412=CARTESIAN_POINT('Ctrl Pts',(0.160821937353092,-0.0493459513256594,
-0.453066666666667));
#25413=CARTESIAN_POINT('Ctrl Pts',(0.15661671770766,-0.0580797720896872,
-0.453066666666667));
#25414=CARTESIAN_POINT('Ctrl Pts',(0.151706204031545,-0.0664127300959662,
-0.453066666666667));
#25415=CARTESIAN_POINT('Ctrl Pts',(0.148524313608442,-0.0718122791095982,
-0.453066666666667));
#25416=CARTESIAN_POINT('Ctrl Pts',(0.145045835105011,-0.0770432405818312,
-0.453066666666667));
#25417=CARTESIAN_POINT('Ctrl Pts',(0.141281936888369,-0.0820744584948006,
-0.453066666666667));
#25418=CARTESIAN_POINT('Ctrl Pts',(0.138548339780333,-0.0857284687642547,
-0.453066666666667));
#25419=CARTESIAN_POINT('Ctrl Pts',(0.135660987987668,-0.0892799913913371,
-0.453066666666667));
#25420=CARTESIAN_POINT('Ctrl Pts',(0.132642788533104,-0.092695561292154,
-0.453066666666667));
#25421=CARTESIAN_POINT('Ctrl Pts',(0.125505940850058,-0.100772032877247,
-0.453066666666667));
#25422=CARTESIAN_POINT('Ctrl Pts',(0.117623386795444,-0.108115570666922,
-0.453066666666667));
#25423=CARTESIAN_POINT('Ctrl Pts',(0.109060973524496,-0.114571708227664,
-0.453066666666667));
#25424=CARTESIAN_POINT('Ctrl Pts',(0.103146709058551,-0.119031117479996,
-0.453066666666667));
#25425=CARTESIAN_POINT('Ctrl Pts',(0.096907460496945,-0.123066412220614,
-0.453066666666667));
#25426=CARTESIAN_POINT('Ctrl Pts',(0.0903606778650195,-0.126612599672284,
-0.453066666666667));
#25427=CARTESIAN_POINT('Origin',(0.,0.,-0.453066666666667));
#25428=CARTESIAN_POINT('Origin',(0.,0.,-0.582472289227037));
#25429=CARTESIAN_POINT('Ctrl Pts',(0.0903606778650195,-0.126612599672284,
-0.453066666666667));
#25430=CARTESIAN_POINT('Ctrl Pts',(0.13200120501619,-0.0968946547775781,
-0.449402649797611));
#25431=CARTESIAN_POINT('Ctrl Pts',(0.183022071105112,0.00628961186891934,
-0.442074616059498));
#25432=CARTESIAN_POINT('Ctrl Pts',(0.0955251259476364,0.156432482487892,
-0.431082565452332));
#25433=CARTESIAN_POINT('Ctrl Pts',(-0.0777334665521386,0.165810192362521,
-0.420090514845164));
#25434=CARTESIAN_POINT('Ctrl Pts',(-0.15183132427248,0.0661923464710166,
-0.412220422770065));
#25435=CARTESIAN_POINT('Ctrl Pts',(-0.155733436132797,0.00767225655067851,
-0.408014347564023));
#25436=CARTESIAN_POINT('Ctrl Pts',(-0.155671978531511,0.000121856215612291,
-0.407472289227037));
#25437=CARTESIAN_POINT('Ctrl Pts',(0.113509973994373,-0.159049193030951,
-0.476074074893873));
#25438=CARTESIAN_POINT('Ctrl Pts',(0.165818292897225,-0.121717875561163,
-0.472410058024817));
#25439=CARTESIAN_POINT('Ctrl Pts',(0.229910078392407,0.00790093319952896,
-0.465082024286706));
#25440=CARTESIAN_POINT('Ctrl Pts',(0.119997490261448,0.196508563665278,
-0.454089973679538));
#25441=CARTESIAN_POINT('Ctrl Pts',(-0.0976478261927854,0.208288727660795,
-0.443097923072371));
#25442=CARTESIAN_POINT('Ctrl Pts',(-0.227652540681624,0.033509185963427,
-0.432105872465202));
#25443=CARTESIAN_POINT('Ctrl Pts',(-0.153475136057457,-0.171473007722053,
-0.421113821858035));
#25444=CARTESIAN_POINT('Ctrl Pts',(0.058385281197714,-0.222565815265022,
-0.410121771250867));
#25445=CARTESIAN_POINT('Ctrl Pts',(0.217866153667128,-0.0740531899532077,
-0.3991297206437));
#25446=CARTESIAN_POINT('Ctrl Pts',(0.181921442653058,0.140906976839248,
-0.388137670036532));
#25447=CARTESIAN_POINT('Ctrl Pts',(-0.0172115249937917,0.229460586201424,
-0.377145619429364));
#25448=CARTESIAN_POINT('Ctrl Pts',(-0.200904477330819,0.112190212191809,
-0.366153568822197));
#25449=CARTESIAN_POINT('Ctrl Pts',(-0.204383566249596,-0.105719475415542,
-0.35516151821503));
#25450=CARTESIAN_POINT('Ctrl Pts',(-0.0245271865868318,-0.228795615786734,
-0.344169467607861));
#25451=CARTESIAN_POINT('Ctrl Pts',(0.17733030957008,-0.146639399315481,
-0.333177417000694));
#25452=CARTESIAN_POINT('Ctrl Pts',(0.220119877306813,0.0670550326110528,
-0.322185366393526));
#25453=CARTESIAN_POINT('Ctrl Pts',(0.0654585025290842,0.220599848939463,
-0.311193315786359));
#25454=CARTESIAN_POINT('Ctrl Pts',(-0.147920131106237,0.176263338113089,
-0.300201265179191));
#25455=CARTESIAN_POINT('Ctrl Pts',(-0.228612151540578,-0.0261841492109524,
-0.289209214572024));
#25456=CARTESIAN_POINT('Ctrl Pts',(-0.104235563843226,-0.205144021139667,
-0.278217163964855));
#25457=CARTESIAN_POINT('Ctrl Pts',(0.113641919270494,-0.200086580128886,
-0.267225113357689));
#25458=CARTESIAN_POINT('Ctrl Pts',(0.229580860068318,-0.0155484015533772,
-0.25623306275052));
#25459=CARTESIAN_POINT('Ctrl Pts',(0.139582253066502,0.182936925549361,
-0.245241012143353));
#25460=CARTESIAN_POINT('Ctrl Pts',(-0.0756237771828058,0.217325032354213,
-0.234248961536185));
#25461=CARTESIAN_POINT('Ctrl Pts',(-0.222994113150184,0.0567692494175366,
-0.223256910929018));
#25462=CARTESIAN_POINT('Ctrl Pts',(-0.170335327486915,-0.154709410547125,
-0.21226486032185));
#25463=CARTESIAN_POINT('Ctrl Pts',(0.0351168847121239,-0.227411376050915,
-0.201272809714682));
#25464=CARTESIAN_POINT('Ctrl Pts',(0.209068659861852,-0.0961218204625421,
-0.190280759107515));
#25465=CARTESIAN_POINT('Ctrl Pts',(0.195482745804626,0.121390419213048,
-0.179288708500347));
#25466=CARTESIAN_POINT('Ctrl Pts',(0.00654561884687529,0.230013710456001,
-0.168296657893179));
#25467=CARTESIAN_POINT('Ctrl Pts',(-0.188262656682081,0.132310954890747,
-0.157304607286012));
#25468=CARTESIAN_POINT('Ctrl Pts',(-0.214197154491775,-0.084076326291454,
-0.146312556678844));
#25469=CARTESIAN_POINT('Ctrl Pts',(-0.0479921676516633,-0.225046671975632,
-0.135320506071676));
#25470=CARTESIAN_POINT('Ctrl Pts',(0.161259941744669,-0.164145144311427,
-0.124328455464509));
#25471=CARTESIAN_POINT('Ctrl Pts',(0.225864351711379,0.0439941137533673,
-0.113336404857341));
#25472=CARTESIAN_POINT('Ctrl Pts',(0.0878555482932161,0.21267566501613,
-0.102344354250174));
#25473=CARTESIAN_POINT('Ctrl Pts',(-0.128943026450155,0.190573028298851,
-0.0913523036430059));
#25474=CARTESIAN_POINT('Ctrl Pts',(-0.23011210049696,-0.00245580332655646,
-0.0803602530358383));
#25475=CARTESIAN_POINT('Ctrl Pts',(-0.124801453245953,-0.193321344114994,
-0.0693682024286707));
#25476=CARTESIAN_POINT('Ctrl Pts',(0.0923324593003295,-0.21069885854053,
-0.058376151821503));
#25477=CARTESIAN_POINT('Ctrl Pts',(0.226884502025437,-0.0392229015181954,
-0.0473841012143354));
#25478=CARTESIAN_POINT('Ctrl Pts',(0.157437865274698,0.167733084004237,
-0.0363920506071677));
#25479=CARTESIAN_POINT('Ctrl Pts',(0.0177060669358754,0.204932776012367,
-0.029064016869056));
#25480=CARTESIAN_POINT('Ctrl Pts',(-0.044842238767986,0.190184998415424,
-0.0254000000000001));
#25481=CARTESIAN_POINT('Ctrl Pts',(0.105793541951255,-0.148236995244729,
-0.468404938818138));
#25482=CARTESIAN_POINT('Ctrl Pts',(0.154545930270213,-0.113443468633301,
-0.464740921949082));
#25483=CARTESIAN_POINT('Ctrl Pts',(0.214280742629976,0.0073638260893257,
-0.457412888210969));
#25484=CARTESIAN_POINT('Ctrl Pts',(0.111840035490177,0.183149869939482,
-0.446420837603803));
#25485=CARTESIAN_POINT('Ctrl Pts',(-0.0910097063125696,0.194129215894703,
-0.435428786996635));
#25486=CARTESIAN_POINT('Ctrl Pts',(-0.212176672810313,0.0312312244133713,
-0.424436736389467));
#25487=CARTESIAN_POINT('Ctrl Pts',(-0.143041863843383,-0.159816236385096,
-0.413444685782299));
#25488=CARTESIAN_POINT('Ctrl Pts',(0.0544162374315441,-0.207435744063536,
-0.402452635175132));
#25489=CARTESIAN_POINT('Ctrl Pts',(0.203055566455196,-0.0690190384355763,
-0.391460584567964));
#25490=CARTESIAN_POINT('Ctrl Pts',(0.169554384499314,0.131328090747395,
-0.380468533960797));
#25491=CARTESIAN_POINT('Ctrl Pts',(-0.0160414818839274,0.213861807013218,
-0.369476483353629));
#25492=CARTESIAN_POINT('Ctrl Pts',(-0.187246948464164,0.104563497835201,
-0.358484432746461));
#25493=CARTESIAN_POINT('Ctrl Pts',(-0.190489528182304,-0.0985326431137525,
-0.347492382139294));
#25494=CARTESIAN_POINT('Ctrl Pts',(-0.0228598232543762,-0.213242041427981,
-0.336500331532126));
#25495=CARTESIAN_POINT('Ctrl Pts',(0.165275357614488,-0.136670821931104,
-0.325508280924959));
#25496=CARTESIAN_POINT('Ctrl Pts',(0.20515608148512,0.0624966173098753,
-0.314516230317791));
#25497=CARTESIAN_POINT('Ctrl Pts',(0.0610086196805955,0.205603424544653,
-0.303524179710623));
#25498=CARTESIAN_POINT('Ctrl Pts',(-0.137864489303809,0.164280919102842,
-0.292532129103455));
#25499=CARTESIAN_POINT('Ctrl Pts',(-0.213071049120087,-0.0244041452088094,
-0.281540078496289));
#25500=CARTESIAN_POINT('Ctrl Pts',(-0.0971496081640168,-0.191198287188087,
-0.27054802788912));
#25501=CARTESIAN_POINT('Ctrl Pts',(0.105916517559595,-0.18648465208703,
-0.259555977281953));
#25502=CARTESIAN_POINT('Ctrl Pts',(0.213973904637198,-0.0144914179267953,
-0.248563926674785));
#25503=CARTESIAN_POINT('Ctrl Pts',(0.130093421976942,0.17050083465352,-0.237571876067617));
#25504=CARTESIAN_POINT('Ctrl Pts',(-0.0704828568130779,0.202551230683597,
-0.22657982546045));
#25505=CARTESIAN_POINT('Ctrl Pts',(-0.207834926167865,0.0529100638336251,
-0.215587774853282));
#25506=CARTESIAN_POINT('Ctrl Pts',(-0.158755895893,-0.144192232092156,-0.204595724246115));
#25507=CARTESIAN_POINT('Ctrl Pts',(0.0327296314610529,-0.211951902602213,
-0.193603673638947));
#25508=CARTESIAN_POINT('Ctrl Pts',(0.194856128139752,-0.089587438774667,
-0.182611623031779));
#25509=CARTESIAN_POINT('Ctrl Pts',(0.182193787393991,0.113138272836999,
-0.171619572424612));
#25510=CARTESIAN_POINT('Ctrl Pts',(0.00610064629305708,0.214377329763965,
-0.160627521817444));
#25511=CARTESIAN_POINT('Ctrl Pts',(-0.175464521457276,0.123316428189286,
-0.149635471210276));
#25512=CARTESIAN_POINT('Ctrl Pts',(-0.199635986619893,-0.0783607998453362,
-0.138643420603109));
#25513=CARTESIAN_POINT('Ctrl Pts',(-0.0447296499428285,-0.209747951610178,
-0.127651369995941));
#25514=CARTESIAN_POINT('Ctrl Pts',(0.150297456793245,-0.152986522679202,
-0.116659319388773));
#25515=CARTESIAN_POINT('Ctrl Pts',(0.210510045304524,0.0410033845942554,
-0.105667268781606));
#25516=CARTESIAN_POINT('Ctrl Pts',(0.0818831095359919,0.198217928320646,
-0.094675218174438));
#25517=CARTESIAN_POINT('Ctrl Pts',(-0.120177452236511,0.177617833522821,
-0.0836831675672705));
#25518=CARTESIAN_POINT('Ctrl Pts',(-0.214469031229127,-0.00228885729693681,
-0.0726911169601027));
#25519=CARTESIAN_POINT('Ctrl Pts',(-0.116317424054805,-0.180179318248426,
-0.0616990663529351));
#25520=CARTESIAN_POINT('Ctrl Pts',(0.0860556791858326,-0.196375505567415,
-0.0507070157457676));
#25521=CARTESIAN_POINT('Ctrl Pts',(0.211460845584438,-0.0365565203760934,
-0.0397149651385997));
#25522=CARTESIAN_POINT('Ctrl Pts',(0.146735205890193,0.156330553472731,
-0.0287229145314322));
#25523=CARTESIAN_POINT('Ctrl Pts',(0.0165024047601763,0.191001402549226,
-0.0213948807933204));
#25524=CARTESIAN_POINT('Ctrl Pts',(-0.0417938538909745,0.17725618199295,
-0.0177308639242646));
#25525=CARTESIAN_POINT('Ctrl Pts',(0.0980771099081373,-0.137424797458507,
-0.460735802742402));
#25526=CARTESIAN_POINT('Ctrl Pts',(0.143273567643201,-0.10516906170544,
-0.457071785873346));
#25527=CARTESIAN_POINT('Ctrl Pts',(0.198651406867544,0.00682671897912246,
-0.449743752135235));
#25528=CARTESIAN_POINT('Ctrl Pts',(0.103682580718907,0.169791176213687,
-0.438751701528067));
#25529=CARTESIAN_POINT('Ctrl Pts',(-0.0843715864323541,0.179969704128612,
-0.427759650920899));
#25530=CARTESIAN_POINT('Ctrl Pts',(-0.196700804939001,0.0289532628633155,
-0.416767600313732));
#25531=CARTESIAN_POINT('Ctrl Pts',(-0.13260859162931,-0.14815946504814,
-0.405775549706564));
#25532=CARTESIAN_POINT('Ctrl Pts',(0.0504471936653742,-0.19230567286205,
-0.394783499099397));
#25533=CARTESIAN_POINT('Ctrl Pts',(0.188244979243263,-0.0639848869179451,
-0.383791448492229));
#25534=CARTESIAN_POINT('Ctrl Pts',(0.157187326345571,0.121749204655543,
-0.372799397885061));
#25535=CARTESIAN_POINT('Ctrl Pts',(-0.014871438774063,0.198263027825011,
-0.361807347277894));
#25536=CARTESIAN_POINT('Ctrl Pts',(-0.17358941959751,0.0969367834785928,
-0.350815296670726));
#25537=CARTESIAN_POINT('Ctrl Pts',(-0.176595490115013,-0.0913458108119624,
-0.339823246063559));
#25538=CARTESIAN_POINT('Ctrl Pts',(-0.021192459921921,-0.197688467069228,
-0.328831195456391));
#25539=CARTESIAN_POINT('Ctrl Pts',(0.153220405658898,-0.126702244546726,
-0.317839144849223));
#25540=CARTESIAN_POINT('Ctrl Pts',(0.190192285663426,0.0579382020086975,
-0.306847094242056));
#25541=CARTESIAN_POINT('Ctrl Pts',(0.056558736832107,0.190607000149843,
-0.295855043634888));
#25542=CARTESIAN_POINT('Ctrl Pts',(-0.127808847501381,0.152298500092595,
-0.28486299302772));
#25543=CARTESIAN_POINT('Ctrl Pts',(-0.197529946699595,-0.0226241412066662,
-0.273870942420553));
#25544=CARTESIAN_POINT('Ctrl Pts',(-0.090063652484807,-0.177252553236508,
-0.262878891813384));
#25545=CARTESIAN_POINT('Ctrl Pts',(0.0981911158486954,-0.172882724045174,
-0.251886841206217));
#25546=CARTESIAN_POINT('Ctrl Pts',(0.198366949206078,-0.0134344343002136,
-0.240894790599049));
#25547=CARTESIAN_POINT('Ctrl Pts',(0.120604590887382,0.158064743757679,
-0.229902739991882));
#25548=CARTESIAN_POINT('Ctrl Pts',(-0.0653419364433495,0.18777742901298,
-0.218910689384714));
#25549=CARTESIAN_POINT('Ctrl Pts',(-0.192675739185548,0.0490508782497135,
-0.207918638777546));
#25550=CARTESIAN_POINT('Ctrl Pts',(-0.147176464299083,-0.133675053637187,
-0.196926588170379));
#25551=CARTESIAN_POINT('Ctrl Pts',(0.0303423782099813,-0.196492429153511,
-0.185934537563211));
#25552=CARTESIAN_POINT('Ctrl Pts',(0.180643596417653,-0.0830530570867919,
-0.174942486956044));
#25553=CARTESIAN_POINT('Ctrl Pts',(0.168904828983355,0.10488612646095,-0.163950436348876));
#25554=CARTESIAN_POINT('Ctrl Pts',(0.00565567373923916,0.198740949071929,
-0.152958385741709));
#25555=CARTESIAN_POINT('Ctrl Pts',(-0.16266638623247,0.114321901487825,
-0.14196633513454));
#25556=CARTESIAN_POINT('Ctrl Pts',(-0.185074818748011,-0.0726452733992181,
-0.130974284527373));
#25557=CARTESIAN_POINT('Ctrl Pts',(-0.0414671322339938,-0.194449231244725,
-0.119982233920205));
#25558=CARTESIAN_POINT('Ctrl Pts',(0.13933497184182,-0.141827901046976,
-0.108990183313038));
#25559=CARTESIAN_POINT('Ctrl Pts',(0.195155738897669,0.038012655435143,
-0.0979981327058701));
#25560=CARTESIAN_POINT('Ctrl Pts',(0.0759106707787678,0.183760191625162,
-0.0870060820987027));
#25561=CARTESIAN_POINT('Ctrl Pts',(-0.111411878022866,0.164662638746789,
-0.0760140314915348));
#25562=CARTESIAN_POINT('Ctrl Pts',(-0.198825961961294,-0.00212191126731689,
-0.0650219808843673));
#25563=CARTESIAN_POINT('Ctrl Pts',(-0.107833394863656,-0.167037292381857,
-0.0540299302771995));
#25564=CARTESIAN_POINT('Ctrl Pts',(0.0797788990713359,-0.1820521525943,
-0.043037879670032));
#25565=CARTESIAN_POINT('Ctrl Pts',(0.196037189143439,-0.0338901392339913,
-0.0320458290628643));
#25566=CARTESIAN_POINT('Ctrl Pts',(0.136032546505688,0.144928022941225,
-0.0210537784556966));
#25567=CARTESIAN_POINT('Ctrl Pts',(0.0152987425844774,0.177070029086086,
-0.0137257447175849));
#25568=CARTESIAN_POINT('Ctrl Pts',(-0.038745469013963,0.164327365570475,
-0.010061727848529));
#25569=CARTESIAN_POINT('Ctrl Pts',(0.0903606778650195,-0.126612599672284,
-0.453066666666667));
#25570=CARTESIAN_POINT('Ctrl Pts',(0.13200120501619,-0.0968946547775781,
-0.449402649797611));
#25571=CARTESIAN_POINT('Ctrl Pts',(0.183022071105112,0.00628961186891934,
-0.442074616059498));
#25572=CARTESIAN_POINT('Ctrl Pts',(0.0955251259476364,0.156432482487892,
-0.431082565452332));
#25573=CARTESIAN_POINT('Ctrl Pts',(-0.0777334665521386,0.165810192362521,
-0.420090514845164));
#25574=CARTESIAN_POINT('Ctrl Pts',(-0.18122493706769,0.0266753013132598,
-0.409098464237996));
#25575=CARTESIAN_POINT('Ctrl Pts',(-0.122175319415237,-0.136502693711184,
-0.398106413630829));
#25576=CARTESIAN_POINT('Ctrl Pts',(0.0464781498992043,-0.177175601660564,
-0.38711436302366));
#25577=CARTESIAN_POINT('Ctrl Pts',(0.17343439203133,-0.0589507354003139,
-0.376122312416494));
#25578=CARTESIAN_POINT('Ctrl Pts',(0.144820268191827,0.112170318563691,
-0.365130261809325));
#25579=CARTESIAN_POINT('Ctrl Pts',(-0.0137013956641988,0.182664248636804,
-0.354138211202158));
#25580=CARTESIAN_POINT('Ctrl Pts',(-0.159931890730855,0.0893100691219848,
-0.34314616059499));
#25581=CARTESIAN_POINT('Ctrl Pts',(-0.162701452047721,-0.0841589785101726,
-0.332154109987823));
#25582=CARTESIAN_POINT('Ctrl Pts',(-0.0195250965894654,-0.182134892710474,
-0.321162059380655));
#25583=CARTESIAN_POINT('Ctrl Pts',(0.141165453703306,-0.116733667162349,
-0.310170008773487));
#25584=CARTESIAN_POINT('Ctrl Pts',(0.175228489841733,0.0533797867075198,
-0.29917795816632));
#25585=CARTESIAN_POINT('Ctrl Pts',(0.052108853983618,0.175610575755033,
-0.288185907559152));
#25586=CARTESIAN_POINT('Ctrl Pts',(-0.117753205698952,0.140316081082348,
-0.277193856951985));
#25587=CARTESIAN_POINT('Ctrl Pts',(-0.181988844279104,-0.0208441372045229,
-0.266201806344817));
#25588=CARTESIAN_POINT('Ctrl Pts',(-0.0829776968055973,-0.163306819284929,
-0.255209755737649));
#25589=CARTESIAN_POINT('Ctrl Pts',(0.0904657141377962,-0.159280796003317,
-0.244217705130481));
#25590=CARTESIAN_POINT('Ctrl Pts',(0.182759993774958,-0.0123774506736319,
-0.233225654523314));
#25591=CARTESIAN_POINT('Ctrl Pts',(0.111115759797821,0.145628652861839,
-0.222233603916146));
#25592=CARTESIAN_POINT('Ctrl Pts',(-0.0602010160736213,0.173003627342364,
-0.211241553308979));
#25593=CARTESIAN_POINT('Ctrl Pts',(-0.17751655220323,0.045191692665802,
-0.200249502701811));
#25594=CARTESIAN_POINT('Ctrl Pts',(-0.135597032705167,-0.123157875182218,
-0.189257452094644));
#25595=CARTESIAN_POINT('Ctrl Pts',(0.0279551249589101,-0.181032955704809,
-0.178265401487475));
#25596=CARTESIAN_POINT('Ctrl Pts',(0.166431064695553,-0.0765186753989169,
-0.167273350880308));
#25597=CARTESIAN_POINT('Ctrl Pts',(0.15561587057272,0.0966339800849018,
-0.15628130027314));
#25598=CARTESIAN_POINT('Ctrl Pts',(0.00521070118542118,0.183104568379892,
-0.145289249665973));
#25599=CARTESIAN_POINT('Ctrl Pts',(-0.149868251007665,0.105327374786364,
-0.134297199058805));
#25600=CARTESIAN_POINT('Ctrl Pts',(-0.170513650876129,-0.0669297469531004,
-0.123305148451637));
#25601=CARTESIAN_POINT('Ctrl Pts',(-0.038204614525159,-0.179150510879271,
-0.11231309784447));
#25602=CARTESIAN_POINT('Ctrl Pts',(0.128372486890396,-0.130669279414751,
-0.101321047237302));
#25603=CARTESIAN_POINT('Ctrl Pts',(0.179801432490814,0.0350219262760309,
-0.0903289966301345));
#25604=CARTESIAN_POINT('Ctrl Pts',(0.0699382320215437,0.169302454929678,
-0.0793369460229671));
#25605=CARTESIAN_POINT('Ctrl Pts',(-0.102646303809221,0.151707443970759,
-0.0683448954157993));
#25606=CARTESIAN_POINT('Ctrl Pts',(-0.18318289269346,-0.00195496523769697,
-0.0573528448086317));
#25607=CARTESIAN_POINT('Ctrl Pts',(-0.0993493656725074,-0.153895266515289,
-0.0463607942014641));
#25608=CARTESIAN_POINT('Ctrl Pts',(0.0735021189568392,-0.167728799621184,
-0.0353687435942965));
#25609=CARTESIAN_POINT('Ctrl Pts',(0.18061353270244,-0.0312237580918893,
-0.0243766929871287));
#25610=CARTESIAN_POINT('Ctrl Pts',(0.125329887121183,0.133525492409719,
-0.0133846423799611));
#25611=CARTESIAN_POINT('Ctrl Pts',(0.0140950804087784,0.163138655622946,
-0.00605660864184936));
#25612=CARTESIAN_POINT('Ctrl Pts',(-0.0356970841369515,0.151398549148,-0.0023925917727935));
#25613=CARTESIAN_POINT('Ctrl Pts',(-0.044842238767986,0.190184998415424,
-0.0254000000000001));
#25614=CARTESIAN_POINT('Ctrl Pts',(0.0177060669358758,0.204932776012367,
-0.029064016869056));
#25615=CARTESIAN_POINT('Ctrl Pts',(0.0875719661052875,0.186332930008301,
-0.0327280337381119));
#25616=CARTESIAN_POINT('Ctrl Pts',(0.13407935514845,0.14254034275253,-0.0363920506071677));
#25617=CARTESIAN_POINT('Ctrl Pts',(0.180586744191612,0.0987477554967585,
-0.0400560674762236));
#25618=CARTESIAN_POINT('Ctrl Pts',(0.203735623108525,0.0297624269892805,
-0.0437200843452796));
#25619=CARTESIAN_POINT('Ctrl Pts',(0.192884722112796,-0.0333095634348471,
-0.0473841012143354));
#25620=CARTESIAN_POINT('Ctrl Pts',(0.182033821117068,-0.0963815538589742,
-0.0510481180833913));
#25621=CARTESIAN_POINT('Ctrl Pts',(0.137183140208699,-0.153540206199751,
-0.0547121349524471));
#25622=CARTESIAN_POINT('Ctrl Pts',(0.0785688143301349,-0.179223279965884,
-0.0583761518215029));
#25623=CARTESIAN_POINT('Ctrl Pts',(0.0199544884515696,-0.204906353732018,
-0.0620401686905588));
#25624=CARTESIAN_POINT('Ctrl Pts',(-0.0524234823971925,-0.199113848923506,
-0.0657041855596148));
#25625=CARTESIAN_POINT('Ctrl Pts',(-0.106164242363408,-0.16440667305451,
-0.0693682024286707));
#25626=CARTESIAN_POINT('Ctrl Pts',(-0.159905002329622,-0.129699497185515,
-0.0730322192977266));
#25627=CARTESIAN_POINT('Ctrl Pts',(-0.195008551413291,-0.0660776502560358,
-0.0766962361667824));
#25628=CARTESIAN_POINT('Ctrl Pts',(-0.195698813613992,-0.00209525485372862,
-0.0803602530358383));
#25629=CARTESIAN_POINT('Ctrl Pts',(-0.195706314304269,-0.00139999422583294,
-0.0804000678419734));
#25630=CARTESIAN_POINT('Ctrl Pts',(-0.195709751492929,-0.000704691024575797,
-0.0804398826481084));
#25631=CARTESIAN_POINT('Ctrl Pts',(-0.195709144608334,-9.38226522190222E-6,
-0.0804796974542435));
#25632=CARTESIAN_POINT('Origin',(0.,0.,-0.199));
#25633=CARTESIAN_POINT('',(0.0577350269189626,-0.1,-0.199));
#25634=CARTESIAN_POINT('',(-0.0577350269189627,-0.1,-0.199));
#25635=CARTESIAN_POINT('',(0.0288675134594813,-0.1,-0.199));
#25636=CARTESIAN_POINT('Origin',(0.,0.,-0.199));
#25637=CARTESIAN_POINT('Origin',(0.,0.,-0.199));
#25638=CARTESIAN_POINT('',(-0.115470053837925,2.77555756156289E-17,-0.199));
#25639=CARTESIAN_POINT('',(-0.0721687836487033,-0.075,-0.199));
#25640=CARTESIAN_POINT('Origin',(0.,0.,-0.199));
#25641=CARTESIAN_POINT('Origin',(0.,0.,-0.199));
#25642=CARTESIAN_POINT('',(-0.0577350269189626,0.1,-0.199));
#25643=CARTESIAN_POINT('',(-0.101036297108185,0.025,-0.199));
#25644=CARTESIAN_POINT('Origin',(0.,0.,-0.199));
#25645=CARTESIAN_POINT('Origin',(0.,0.,-0.199));
#25646=CARTESIAN_POINT('',(0.0577350269189626,0.1,-0.199));
#25647=CARTESIAN_POINT('',(-0.0288675134594813,0.1,-0.199));
#25648=CARTESIAN_POINT('Origin',(0.,0.,-0.199));
#25649=CARTESIAN_POINT('Origin',(0.,0.,-0.199));
#25650=CARTESIAN_POINT('',(0.115470053837925,0.,-0.199));
#25651=CARTESIAN_POINT('',(0.0721687836487032,0.075,-0.199));
#25652=CARTESIAN_POINT('Origin',(0.,0.,-0.199));
#25653=CARTESIAN_POINT('Origin',(0.,0.,-0.199));
#25654=CARTESIAN_POINT('',(0.101036297108185,-0.025,-0.199));
#25655=CARTESIAN_POINT('Origin',(0.,0.,-0.199));
#25656=CARTESIAN_POINT('Origin',(0.,0.,-0.234141016151378));
#25657=CARTESIAN_POINT('',(0.,0.,-0.269282032302755));
#25658=CARTESIAN_POINT('',(-0.113827101150665,-1.39397995080384E-17,-0.2));
#25659=CARTESIAN_POINT('',(-0.0577350269189626,-7.07050159149938E-18,-0.234141016151378));
#25660=CARTESIAN_POINT('',(-0.113789894775128,-0.00291012086156119,-0.2));
#25661=CARTESIAN_POINT('Origin',(0.,0.,-0.2));
#25662=CARTESIAN_POINT('Ctrl Pts',(-0.115470053837925,-1.38777878078145E-17,
-0.199));
#25663=CARTESIAN_POINT('Ctrl Pts',(-0.114623954995367,-0.00146548618353618,
-0.199514986736453));
#25664=CARTESIAN_POINT('Ctrl Pts',(-0.113789894775128,-0.00291012086156124,
-0.2));
#25665=CARTESIAN_POINT('',(-0.0594151859817593,-0.0970898791384388,-0.2));
#25666=CARTESIAN_POINT('Ctrl Pts',(-0.0594151859817594,-0.0970898791384387,
-0.2));
#25667=CARTESIAN_POINT('Ctrl Pts',(-0.0585811257615208,-0.0985345138164641,
-0.199514986736453));
#25668=CARTESIAN_POINT('Ctrl Pts',(-0.0577350269189627,-0.1,-0.199));
#25669=CARTESIAN_POINT('',(-0.0543747087933692,-0.1,-0.2));
#25670=CARTESIAN_POINT('Origin',(0.,0.,-0.2));
#25671=CARTESIAN_POINT('Ctrl Pts',(-0.0577350269189627,-0.1,-0.199));
#25672=CARTESIAN_POINT('Ctrl Pts',(-0.0560428292338519,-0.1,-0.199514986736451));
#25673=CARTESIAN_POINT('Ctrl Pts',(-0.0543747087933692,-0.1,-0.2));
#25674=CARTESIAN_POINT('',(0.0543747087933691,-0.1,-0.2));
#25675=CARTESIAN_POINT('Ctrl Pts',(0.0543747087933691,-0.1,-0.2));
#25676=CARTESIAN_POINT('Ctrl Pts',(0.056042829233854,-0.1,-0.19951498673645));
#25677=CARTESIAN_POINT('Ctrl Pts',(0.0577350269189626,-0.1,-0.199));
#25678=CARTESIAN_POINT('',(0.0594151859817594,-0.0970898791384387,-0.2));
#25679=CARTESIAN_POINT('Origin',(0.,0.,-0.2));
#25680=CARTESIAN_POINT('Ctrl Pts',(0.0577350269189626,-0.1,-0.199));
#25681=CARTESIAN_POINT('Ctrl Pts',(0.0585811257615188,-0.0985345138164674,
-0.199514986736451));
#25682=CARTESIAN_POINT('Ctrl Pts',(0.0594151859817594,-0.0970898791384387,
-0.2));
#25683=CARTESIAN_POINT('',(0.113789894775128,-0.00291012086156127,-0.2));
#25684=CARTESIAN_POINT('Ctrl Pts',(0.113789894775128,-0.00291012086156127,
-0.2));
#25685=CARTESIAN_POINT('Ctrl Pts',(0.114623954995369,-0.00146548618353307,
-0.199514986736452));
#25686=CARTESIAN_POINT('Ctrl Pts',(0.115470053837925,1.38777878078145E-17,
-0.199));
#25687=CARTESIAN_POINT('',(0.113789894775128,0.00291012086156127,-0.2));
#25688=CARTESIAN_POINT('Origin',(0.,0.,-0.2));
#25689=CARTESIAN_POINT('Ctrl Pts',(0.115470053837925,0.,-0.199));
#25690=CARTESIAN_POINT('Ctrl Pts',(0.114623954995369,0.00146548618353293,
-0.199514986736452));
#25691=CARTESIAN_POINT('Ctrl Pts',(0.113789894775128,0.00291012086156128,
-0.2));
#25692=CARTESIAN_POINT('',(0.0594151859817593,0.0970898791384387,-0.2));
#25693=CARTESIAN_POINT('Ctrl Pts',(0.0594151859817593,0.0970898791384387,
-0.2));
#25694=CARTESIAN_POINT('Ctrl Pts',(0.0585811257615177,0.0985345138164694,
-0.199514986736451));
#25695=CARTESIAN_POINT('Ctrl Pts',(0.0577350269189626,0.1,-0.199));
#25696=CARTESIAN_POINT('',(0.0543747087933691,0.1,-0.2));
#25697=CARTESIAN_POINT('Origin',(0.,0.,-0.2));
#25698=CARTESIAN_POINT('Ctrl Pts',(0.0577350269189626,0.1,-0.199));
#25699=CARTESIAN_POINT('Ctrl Pts',(0.0560428292338471,0.1,-0.199514986736452));
#25700=CARTESIAN_POINT('Ctrl Pts',(0.0543747087933691,0.1,-0.2));
#25701=CARTESIAN_POINT('',(-0.0543747087933691,0.1,-0.2));
#25702=CARTESIAN_POINT('Ctrl Pts',(-0.0543747087933691,0.1,-0.2));
#25703=CARTESIAN_POINT('Ctrl Pts',(-0.0560428292338464,0.1,-0.199514986736453));
#25704=CARTESIAN_POINT('Ctrl Pts',(-0.0577350269189626,0.1,-0.199));
#25705=CARTESIAN_POINT('',(-0.0594151859817593,0.0970898791384387,-0.2));
#25706=CARTESIAN_POINT('Origin',(0.,0.,-0.2));
#25707=CARTESIAN_POINT('Ctrl Pts',(-0.0577350269189626,0.1,-0.199));
#25708=CARTESIAN_POINT('Ctrl Pts',(-0.0585811257615179,0.0985345138164689,
-0.199514986736451));
#25709=CARTESIAN_POINT('Ctrl Pts',(-0.0594151859817593,0.0970898791384388,
-0.2));
#25710=CARTESIAN_POINT('',(-0.113789894775128,0.0029101208615613,-0.2));
#25711=CARTESIAN_POINT('Ctrl Pts',(-0.113789894775128,0.00291012086156131,
-0.2));
#25712=CARTESIAN_POINT('Ctrl Pts',(-0.11462395499537,0.00146548618353128,
-0.199514986736451));
#25713=CARTESIAN_POINT('Ctrl Pts',(-0.115470053837925,2.08166817117217E-17,
-0.199));
#25714=CARTESIAN_POINT('Origin',(0.,0.,-0.2));
#25715=CARTESIAN_POINT('Origin',(-0.115470053837925,1.38777878078145E-17,
0.));
#25716=CARTESIAN_POINT('',(-0.0577350269189626,0.1,0.));
#25717=CARTESIAN_POINT('',(-0.0577350269189626,0.1,0.));
#25718=CARTESIAN_POINT('',(-0.115470053837925,1.41410031829988E-17,0.));
#25719=CARTESIAN_POINT('',(-0.101036297108185,0.025,0.));
#25720=CARTESIAN_POINT('',(-0.115470053837925,1.41410031829988E-17,0.));
#25721=CARTESIAN_POINT('Origin',(-0.115470053837925,1.38777878078145E-17,
0.));
#25722=CARTESIAN_POINT('',(-0.115470053837925,1.38777878078145E-17,-0.2));
#25723=CARTESIAN_POINT('',(-0.115470053837925,1.41410031829988E-17,0.));
#25724=CARTESIAN_POINT('',(-0.0577350269189626,0.1,-0.2));
#25725=CARTESIAN_POINT('Origin',(-0.0577350269189626,0.1,0.));
#25726=CARTESIAN_POINT('',(0.0577350269189626,0.1,0.));
#25727=CARTESIAN_POINT('',(0.0577350269189626,0.1,0.));
#25728=CARTESIAN_POINT('',(-0.0288675134594813,0.1,0.));
#25729=CARTESIAN_POINT('Origin',(-0.0577350269189626,0.1,0.));
#25730=CARTESIAN_POINT('',(0.0577350269189626,0.1,-0.2));
#25731=CARTESIAN_POINT('',(0.0577350269189626,0.1,-0.2));
#25732=CARTESIAN_POINT('',(0.0577350269189626,0.1,0.));
#25733=CARTESIAN_POINT('Origin',(-0.0577350269189626,0.1,0.));
#25734=CARTESIAN_POINT('',(-0.0577350269189626,0.1,-0.2));
#25735=CARTESIAN_POINT('',(-0.0577350269189626,0.1,0.));
#25736=CARTESIAN_POINT('',(0.0577350269189626,0.1,-0.2));
#25737=CARTESIAN_POINT('Origin',(-0.0577350269189626,-0.1,0.));
#25738=CARTESIAN_POINT('',(-0.0577350269189626,-0.1,0.));
#25739=CARTESIAN_POINT('',(-0.0721687836487033,-0.075,0.));
#25740=CARTESIAN_POINT('',(-0.0577350269189626,-0.1,0.));
#25741=CARTESIAN_POINT('Origin',(-0.0577350269189626,-0.1,0.));
#25742=CARTESIAN_POINT('',(-0.0577350269189626,-0.1,-0.2));
#25743=CARTESIAN_POINT('',(-0.0577350269189626,-0.1,0.));
#25744=CARTESIAN_POINT('',(-0.115470053837925,1.41410031829988E-17,-0.2));
#25745=CARTESIAN_POINT('Origin',(0.0577350269189626,0.1,0.));
#25746=CARTESIAN_POINT('',(0.115470053837925,0.,0.));
#25747=CARTESIAN_POINT('',(0.115470053837925,0.,0.));
#25748=CARTESIAN_POINT('',(0.0721687836487032,0.075,0.));
#25749=CARTESIAN_POINT('Origin',(0.0577350269189626,0.1,0.));
#25750=CARTESIAN_POINT('',(0.115470053837925,0.,-0.2));
#25751=CARTESIAN_POINT('',(0.115470053837925,0.,-0.2));
#25752=CARTESIAN_POINT('',(0.115470053837925,0.,0.));
#25753=CARTESIAN_POINT('Origin',(0.0577350269189626,0.1,0.));
#25754=CARTESIAN_POINT('',(0.115470053837925,0.,-0.2));
#25755=CARTESIAN_POINT('Origin',(0.,0.,-0.2));
#25756=CARTESIAN_POINT('',(-0.0577350269189626,0.1,-0.2));
#25757=CARTESIAN_POINT('Origin',(0.,0.,-0.2));
#25758=CARTESIAN_POINT('Origin',(0.,0.,-0.2));
#25759=CARTESIAN_POINT('',(0.0577350269189626,-0.1,-0.2));
#25760=CARTESIAN_POINT('Origin',(0.,0.,-0.2));
#25761=CARTESIAN_POINT('',(0.0577350269189626,-0.1,-0.2));
#25762=CARTESIAN_POINT('',(-0.0577350269189626,-0.1,-0.2));
#25763=CARTESIAN_POINT('',(0.0577350269189626,-0.1,-0.2));
#25764=CARTESIAN_POINT('Origin',(0.,0.,-0.2));
#25765=CARTESIAN_POINT('',(-0.0577350269189626,-0.1,-0.2));
#25766=CARTESIAN_POINT('Origin',(0.,0.,-0.2));
#25767=CARTESIAN_POINT('',(-0.115470053837925,1.41410031829988E-17,-0.2));
#25768=CARTESIAN_POINT('Origin',(0.115470053837925,0.,0.));
#25769=CARTESIAN_POINT('',(0.0577350269189626,-0.1,0.));
#25770=CARTESIAN_POINT('',(0.0577350269189626,-0.1,0.));
#25771=CARTESIAN_POINT('',(0.101036297108185,-0.025,0.));
#25772=CARTESIAN_POINT('Origin',(0.115470053837925,0.,0.));
#25773=CARTESIAN_POINT('',(0.0577350269189626,-0.1,0.));
#25774=CARTESIAN_POINT('Origin',(0.115470053837925,0.,0.));
#25775=CARTESIAN_POINT('Origin',(0.0577350269189626,-0.1,0.));
#25776=CARTESIAN_POINT('Origin',(0.0577350269189626,-0.1,0.));
#25777=CARTESIAN_POINT('',(0.0288675134594813,-0.1,0.));
#25778=CARTESIAN_POINT('Origin',(-0.115470053837925,1.38777878078145E-17,
0.));
#25779=CARTESIAN_POINT('Origin',(-0.0577350269189626,-0.1,0.));
#25780=CARTESIAN_POINT('Origin',(0.0577350269189626,-0.1,0.));
#25781=CARTESIAN_POINT('Origin',(0.125,0.,-0.5));
#25782=CARTESIAN_POINT('',(-0.125,-1.53080849893419E-17,-0.5));
#25783=CARTESIAN_POINT('Origin',(0.,0.,-0.5));
#25784=CARTESIAN_POINT('Origin',(0.,0.,-0.475));
#25785=CARTESIAN_POINT('',(-0.1625,-1.99005104861445E-17,-0.475));
#25786=CARTESIAN_POINT('Origin',(0.,0.,-0.24));
#25787=CARTESIAN_POINT('Origin',(0.,0.,-0.0254000000000001));
#25788=CARTESIAN_POINT('Origin',(0.,0.,-0.015));
#25789=CARTESIAN_POINT('',(-0.17,-2.0818995585505E-17,-1.73472347597681E-18));
#25790=CARTESIAN_POINT('Origin',(0.,0.,0.));
#25791=CARTESIAN_POINT('',(-0.185,-2.2655965784226E-17,-0.015));
#25792=CARTESIAN_POINT('Origin',(0.,0.,0.));
#38587=UNCERTAINTY_MEASURE_WITH_UNIT(LENGTH_MEASURE(0.001),#38612,
'DISTANCE_ACCURACY_VALUE',
'Maximum model space distance between geometric entities at asserted c
onnectivities');
#38595=UNCERTAINTY_MEASURE_WITH_UNIT(LENGTH_MEASURE(0.001),#38612,
'DISTANCE_ACCURACY_VALUE',
'Maximum model space distance between geometric entities at asserted c
onnectivities');
#38603=(
GEOMETRIC_REPRESENTATION_CONTEXT(3)
GLOBAL_UNCERTAINTY_ASSIGNED_CONTEXT((#38587))
GLOBAL_UNIT_ASSIGNED_CONTEXT((#38612,#38614,#38615))
REPRESENTATION_CONTEXT('','3D')
);
#38611=(
GEOMETRIC_REPRESENTATION_CONTEXT(3)
GLOBAL_UNCERTAINTY_ASSIGNED_CONTEXT((#38595))
GLOBAL_UNIT_ASSIGNED_CONTEXT((#38612,#38614,#38615))
REPRESENTATION_CONTEXT('','3D')
);
#38612=(
LENGTH_UNIT()
NAMED_UNIT(*)
SI_UNIT(.CENTI.,.METRE.)
);
#38614=(
NAMED_UNIT(*)
PLANE_ANGLE_UNIT()
SI_UNIT($,.RADIAN.)
);
#38615=(
NAMED_UNIT(*)
SI_UNIT($,.STERADIAN.)
SOLID_ANGLE_UNIT()
);
#38623=SHAPE_DEFINITION_REPRESENTATION(#38638,#38674);
#38638=PRODUCT_DEFINITION_SHAPE('',$,#38690);
#38674=SHAPE_REPRESENTATION('',(#16834),#38603);
#38682=PRODUCT_DEFINITION_CONTEXT('part definition',#38729,'design');
#38690=PRODUCT_DEFINITION('2026-10-19-02-32-11-430',
'13_ISO_4026_M4x5_Set_Screw',#38705,#38682);
#38705=PRODUCT_DEFINITION_FORMATION('',$,#38738);
#38729=APPLICATION_CONTEXT(
'Core Data for Automotive Mechanical Design Process');
#38730=PRODUCT_CONTEXT('part definition',#38729,'mechanical');
#38738=PRODUCT('2026-10-19-02-32-11-430','13_ISO_4026_M4x5_Set_Screw',$,
(#38730));
#38879=COLOUR_RGB('Black',0.12,0.14,0.17);
#38880=FILL_AREA_STYLE_COLOUR('',#38879);
#38881=FILL_AREA_STYLE('',(#38880));
#38882=SURFACE_STYLE_FILL_AREA(#38881);
#38883=SURFACE_SIDE_STYLE('',(#38882));
#38884=SURFACE_STYLE_USAGE(.BOTH.,#38883);
#38885=PRESENTATION_STYLE_ASSIGNMENT((#38884));
ENDSEC;
END-ISO-10303-21;
